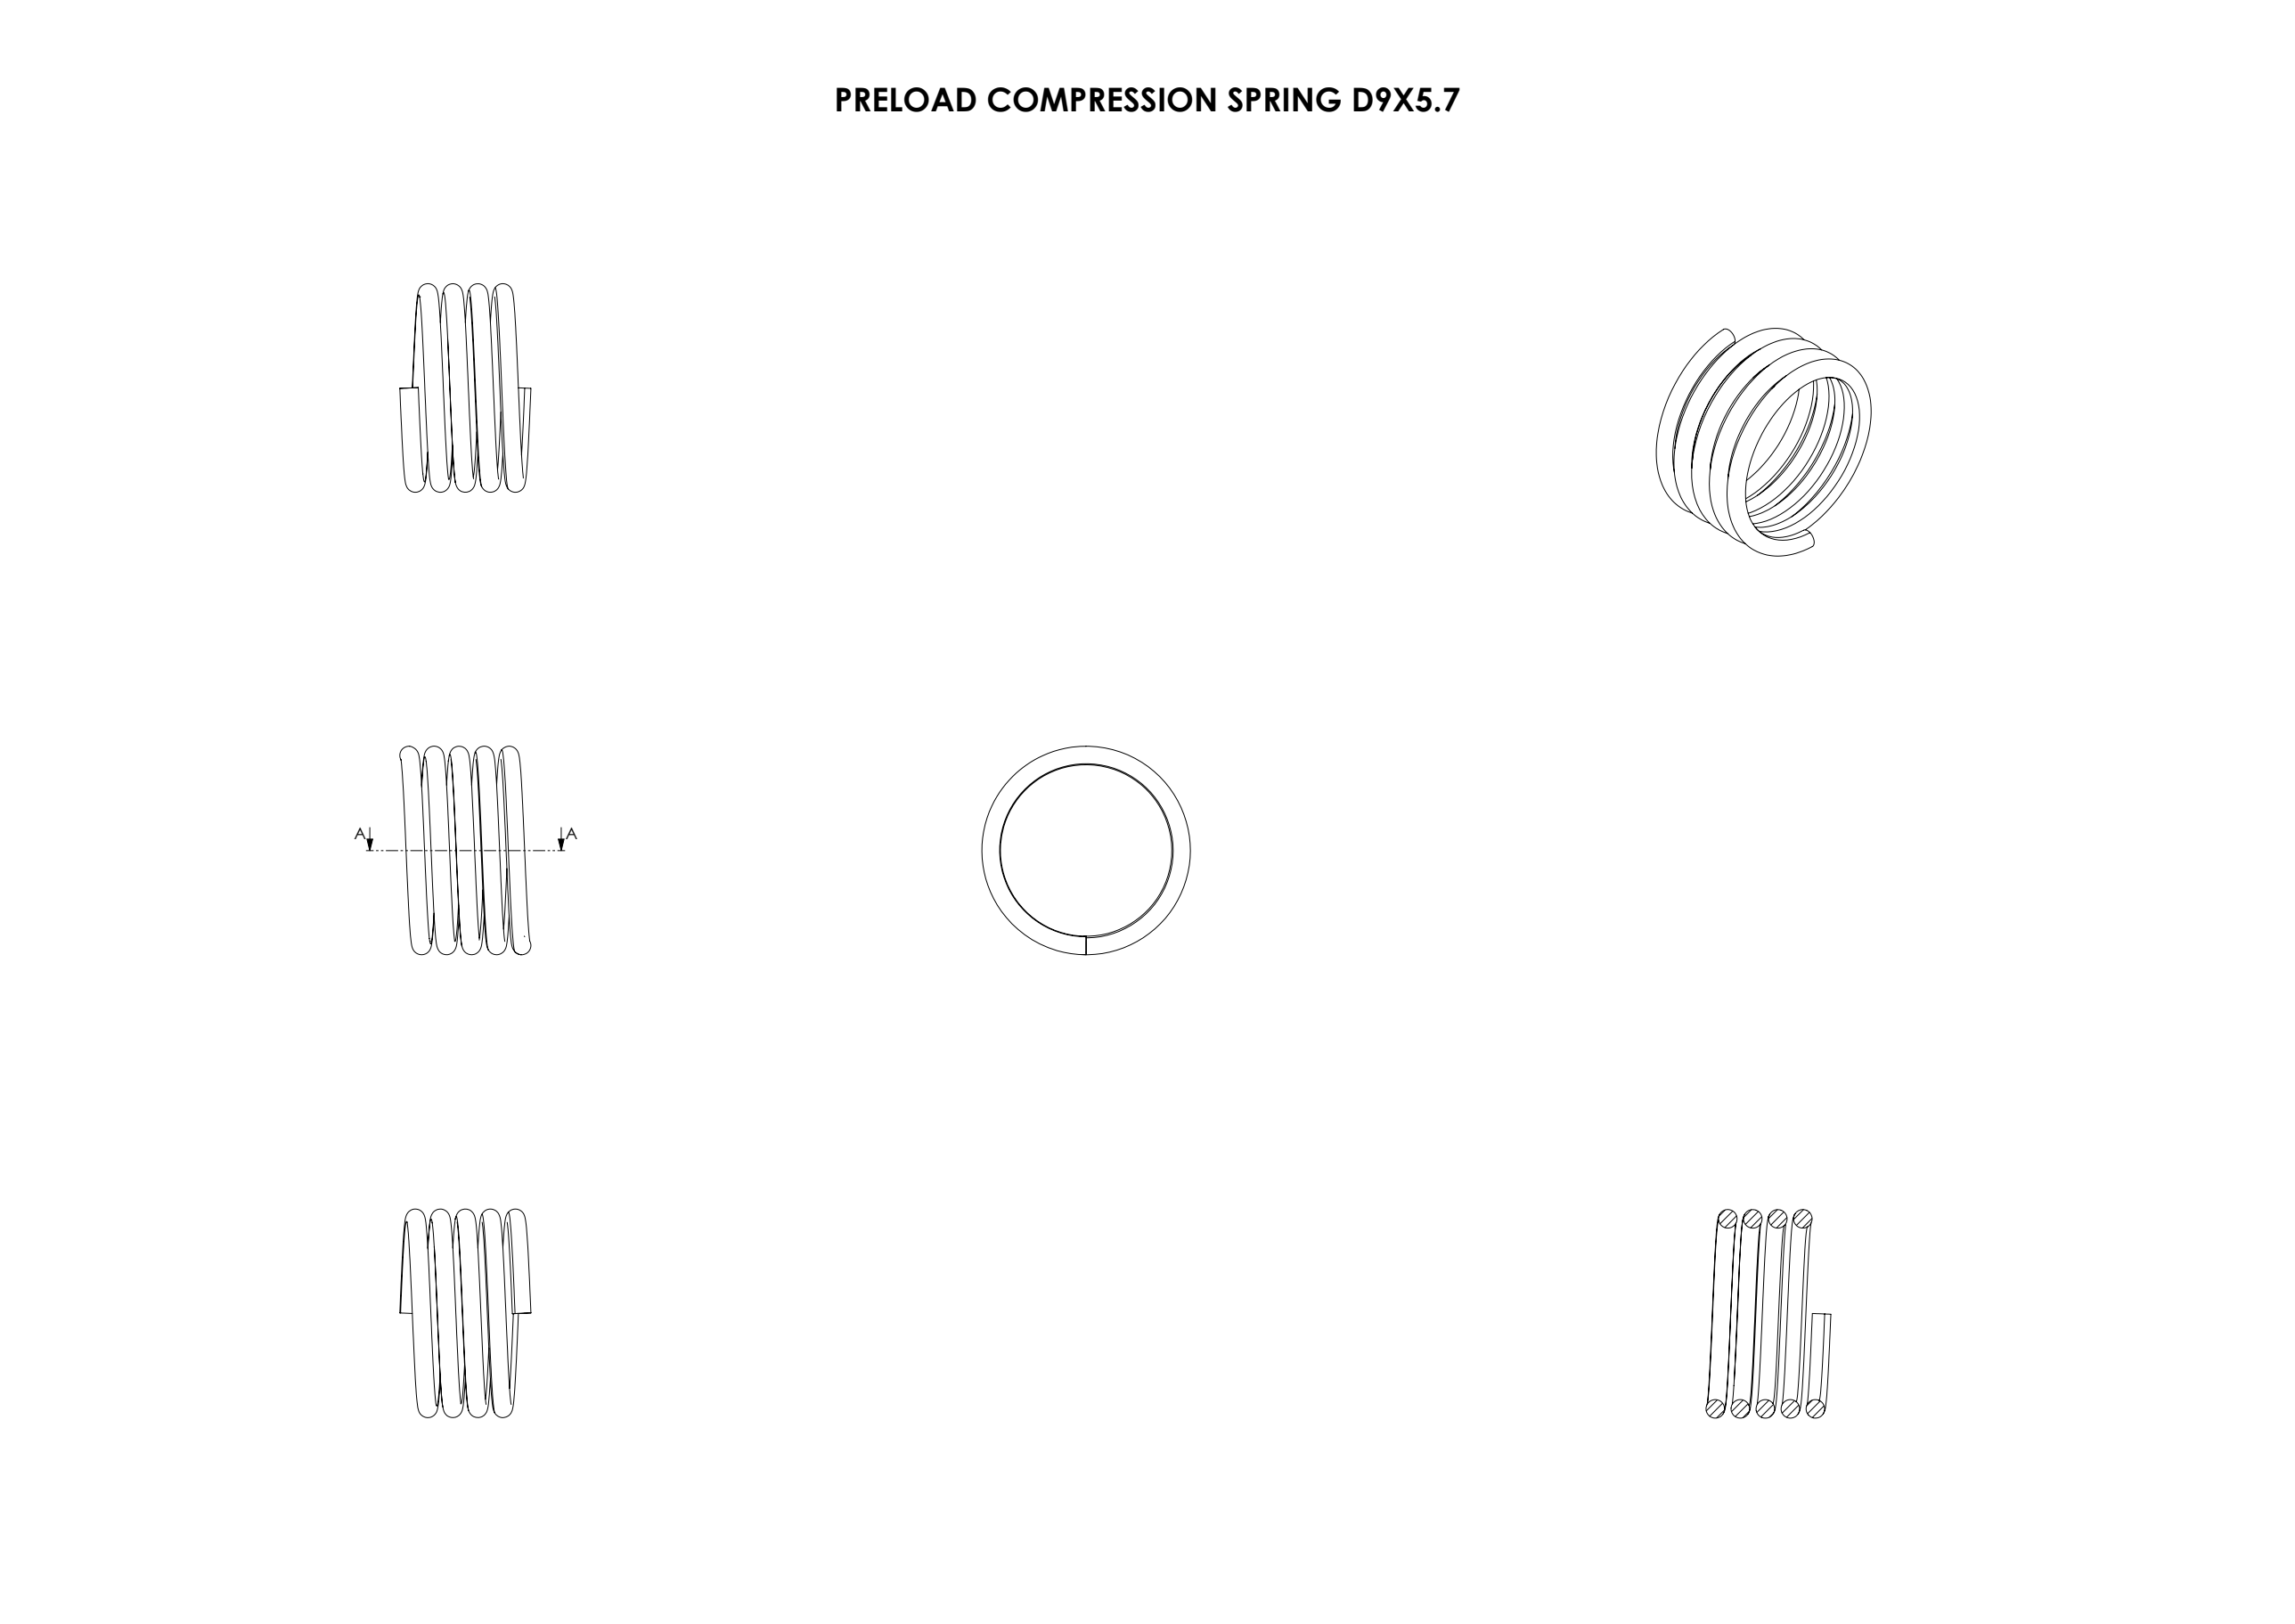
ISO-10303-21;
HEADER;
/* Generated by software containing ST-Developer
 * from STEP Tools, Inc. (www.steptools.com) 
 */

FILE_DESCRIPTION(
/* description */ (''),
/* implementation_level */ '2;1');

FILE_NAME(
/* name */ '13_Preload_Compression_Spring_D9x5.7.step',
/* time_stamp */ '2026-10-21T01:56:51-07:00',
/* author */ (''),
/* organization */ (''),
/* preprocessor_version */ 'ST-DEVELOPER v20.2',
/* originating_system */ 'Autodesk Translation Framework v15.15.0.0',
/* authorisation */ '');

FILE_SCHEMA (('AUTOMOTIVE_DESIGN { 1 0 10303 214 3 1 1 }'));
ENDSEC;

DATA;
#10=MECHANICAL_DESIGN_GEOMETRIC_PRESENTATION_REPRESENTATION('',(#279),#82384);
#241=SHAPE_REPRESENTATION_RELATIONSHIP('SRR','None',#82475,#260);
#260=ADVANCED_BREP_SHAPE_REPRESENTATION('',(#298),#82374);
#279=STYLED_ITEM('',(#82631),#298);
#298=MANIFOLD_SOLID_BREP('Body1',#30670);
#421=B_SPLINE_SURFACE_WITH_KNOTS('',3,3,((#48911,#48912,#48913,#48914,#48915,
#48916,#48917,#48918,#48919,#48920,#48921,#48922,#48923,#48924,#48925,#48926,
#48927,#48928,#48929,#48930,#48931,#48932,#48933,#48934,#48935,#48936,#48937,
#48938,#48939,#48940,#48941,#48942,#48943,#48944,#48945,#48946,#48947,#48948,
#48949,#48950,#48951,#48952,#48953,#48954,#48955,#48956,#48957,#48958,#48959,
#48960,#48961,#48962,#48963,#48964,#48965,#48966,#48967),(#48968,#48969,
#48970,#48971,#48972,#48973,#48974,#48975,#48976,#48977,#48978,#48979,#48980,
#48981,#48982,#48983,#48984,#48985,#48986,#48987,#48988,#48989,#48990,#48991,
#48992,#48993,#48994,#48995,#48996,#48997,#48998,#48999,#49000,#49001,#49002,
#49003,#49004,#49005,#49006,#49007,#49008,#49009,#49010,#49011,#49012,#49013,
#49014,#49015,#49016,#49017,#49018,#49019,#49020,#49021,#49022,#49023,#49024),
(#49025,#49026,#49027,#49028,#49029,#49030,#49031,#49032,#49033,#49034,
#49035,#49036,#49037,#49038,#49039,#49040,#49041,#49042,#49043,#49044,#49045,
#49046,#49047,#49048,#49049,#49050,#49051,#49052,#49053,#49054,#49055,#49056,
#49057,#49058,#49059,#49060,#49061,#49062,#49063,#49064,#49065,#49066,#49067,
#49068,#49069,#49070,#49071,#49072,#49073,#49074,#49075,#49076,#49077,#49078,
#49079,#49080,#49081),(#49082,#49083,#49084,#49085,#49086,#49087,#49088,
#49089,#49090,#49091,#49092,#49093,#49094,#49095,#49096,#49097,#49098,#49099,
#49100,#49101,#49102,#49103,#49104,#49105,#49106,#49107,#49108,#49109,#49110,
#49111,#49112,#49113,#49114,#49115,#49116,#49117,#49118,#49119,#49120,#49121,
#49122,#49123,#49124,#49125,#49126,#49127,#49128,#49129,#49130,#49131,#49132,
#49133,#49134,#49135,#49136,#49137,#49138),(#49139,#49140,#49141,#49142,
#49143,#49144,#49145,#49146,#49147,#49148,#49149,#49150,#49151,#49152,#49153,
#49154,#49155,#49156,#49157,#49158,#49159,#49160,#49161,#49162,#49163,#49164,
#49165,#49166,#49167,#49168,#49169,#49170,#49171,#49172,#49173,#49174,#49175,
#49176,#49177,#49178,#49179,#49180,#49181,#49182,#49183,#49184,#49185,#49186,
#49187,#49188,#49189,#49190,#49191,#49192,#49193,#49194,#49195),(#49196,
#49197,#49198,#49199,#49200,#49201,#49202,#49203,#49204,#49205,#49206,#49207,
#49208,#49209,#49210,#49211,#49212,#49213,#49214,#49215,#49216,#49217,#49218,
#49219,#49220,#49221,#49222,#49223,#49224,#49225,#49226,#49227,#49228,#49229,
#49230,#49231,#49232,#49233,#49234,#49235,#49236,#49237,#49238,#49239,#49240,
#49241,#49242,#49243,#49244,#49245,#49246,#49247,#49248,#49249,#49250,#49251,
#49252),(#49253,#49254,#49255,#49256,#49257,#49258,#49259,#49260,#49261,
#49262,#49263,#49264,#49265,#49266,#49267,#49268,#49269,#49270,#49271,#49272,
#49273,#49274,#49275,#49276,#49277,#49278,#49279,#49280,#49281,#49282,#49283,
#49284,#49285,#49286,#49287,#49288,#49289,#49290,#49291,#49292,#49293,#49294,
#49295,#49296,#49297,#49298,#49299,#49300,#49301,#49302,#49303,#49304,#49305,
#49306,#49307,#49308,#49309),(#49310,#49311,#49312,#49313,#49314,#49315,
#49316,#49317,#49318,#49319,#49320,#49321,#49322,#49323,#49324,#49325,#49326,
#49327,#49328,#49329,#49330,#49331,#49332,#49333,#49334,#49335,#49336,#49337,
#49338,#49339,#49340,#49341,#49342,#49343,#49344,#49345,#49346,#49347,#49348,
#49349,#49350,#49351,#49352,#49353,#49354,#49355,#49356,#49357,#49358,#49359,
#49360,#49361,#49362,#49363,#49364,#49365,#49366),(#49367,#49368,#49369,
#49370,#49371,#49372,#49373,#49374,#49375,#49376,#49377,#49378,#49379,#49380,
#49381,#49382,#49383,#49384,#49385,#49386,#49387,#49388,#49389,#49390,#49391,
#49392,#49393,#49394,#49395,#49396,#49397,#49398,#49399,#49400,#49401,#49402,
#49403,#49404,#49405,#49406,#49407,#49408,#49409,#49410,#49411,#49412,#49413,
#49414,#49415,#49416,#49417,#49418,#49419,#49420,#49421,#49422,#49423),
(#49424,#49425,#49426,#49427,#49428,#49429,#49430,#49431,#49432,#49433,
#49434,#49435,#49436,#49437,#49438,#49439,#49440,#49441,#49442,#49443,#49444,
#49445,#49446,#49447,#49448,#49449,#49450,#49451,#49452,#49453,#49454,#49455,
#49456,#49457,#49458,#49459,#49460,#49461,#49462,#49463,#49464,#49465,#49466,
#49467,#49468,#49469,#49470,#49471,#49472,#49473,#49474,#49475,#49476,#49477,
#49478,#49479,#49480)),.UNSPECIFIED.,.T.,.F.,.F.,(4,1,1,1,1,1,1,4),(4,1,
1,1,1,1,1,1,1,1,1,1,1,1,1,1,1,1,1,1,1,1,1,1,1,1,1,1,1,1,1,1,1,1,1,1,1,1,
1,1,1,1,1,1,1,1,1,1,1,1,1,1,1,1,4),(-3.14159265358979,-2.24399475256414,
-1.34639685153848,-0.448798950512828,0.448798950512828,1.34639685153848,
2.24399475256414,3.14159265358979),(0.,0.00892857142857143,0.0178571428571429,
0.0357142857142857,0.0535714285714286,0.0714285714285714,0.0892857142857143,
0.107142857142857,0.125,0.142857142857143,0.166666666666667,0.19047619047619,
0.214285714285714,0.232142857142857,0.25,0.267857142857143,0.285714285714286,
0.303571428571429,0.321428571428571,0.339285714285714,0.357142857142857,
0.375,0.392857142857143,0.410714285714286,0.428571428571429,0.452380952380952,
0.476190476190476,0.5,0.523809523809524,0.547619047619048,0.571428571428571,
0.595238095238095,0.619047619047619,0.642857142857143,0.666666666666667,
0.682539682539682,0.698412698412698,0.714285714285714,0.73015873015873,
0.746031746031746,0.761904761904762,0.785714285714286,0.809523809523809,
0.833333333333333,0.857142857142857,0.866071428571429,0.875,0.892857142857143,
0.910714285714286,0.928571428571429,0.946428571428571,0.964285714285714,
0.982142857142857,0.991071428571429,1.),.UNSPECIFIED.);
#1533=CIRCLE('',#32089,0.4);
#1534=CIRCLE('',#32090,0.4);
#2374=B_SPLINE_CURVE_WITH_KNOTS('',3,(#49484,#49485,#49486,#49487,#49488,
#49489,#49490,#49491,#49492,#49493,#49494,#49495,#49496,#49497,#49498,#49499,
#49500,#49501,#49502,#49503,#49504,#49505,#49506,#49507,#49508,#49509,#49510,
#49511,#49512,#49513,#49514,#49515,#49516,#49517,#49518,#49519,#49520,#49521,
#49522,#49523,#49524,#49525,#49526,#49527,#49528,#49529,#49530,#49531,#49532,
#49533,#49534,#49535,#49536,#49537,#49538,#49539,#49540),.UNSPECIFIED.,
 .F.,.F.,(4,1,1,1,1,1,1,1,1,1,1,1,1,1,1,1,1,1,1,1,1,1,1,1,1,1,1,1,1,1,1,
1,1,1,1,1,1,1,1,1,1,1,1,1,1,1,1,1,1,1,1,1,1,1,4),(0.,0.00892857142857143,
0.0178571428571429,0.0357142857142857,0.0535714285714286,0.0714285714285714,
0.0892857142857143,0.107142857142857,0.125,0.142857142857143,0.166666666666667,
0.19047619047619,0.214285714285714,0.232142857142857,0.25,0.267857142857143,
0.285714285714286,0.303571428571429,0.321428571428571,0.339285714285714,
0.357142857142857,0.375,0.392857142857143,0.410714285714286,0.428571428571429,
0.452380952380952,0.476190476190476,0.5,0.523809523809524,0.547619047619048,
0.571428571428571,0.595238095238095,0.619047619047619,0.642857142857143,
0.666666666666667,0.682539682539682,0.698412698412698,0.714285714285714,
0.73015873015873,0.746031746031746,0.761904761904762,0.785714285714286,
0.809523809523809,0.833333333333333,0.857142857142857,0.866071428571429,
0.875,0.892857142857143,0.910714285714286,0.928571428571429,0.946428571428571,
0.964285714285714,0.982142857142857,0.991071428571429,1.),.UNSPECIFIED.);
#4381=FACE_OUTER_BOUND('',#6339,.T.);
#4382=FACE_OUTER_BOUND('',#6340,.T.);
#4383=FACE_OUTER_BOUND('',#6341,.T.);
#6339=EDGE_LOOP('',(#23055,#23056,#23057,#23058));
#6340=EDGE_LOOP('',(#23059));
#6341=EDGE_LOOP('',(#23060));
#13185=VERTEX_POINT('',#49481);
#13186=VERTEX_POINT('',#49483);
#16749=EDGE_CURVE('',#13185,#13185,#1533,.T.);
#16750=EDGE_CURVE('',#13185,#13186,#2374,.T.);
#16751=EDGE_CURVE('',#13186,#13186,#1534,.T.);
#23055=ORIENTED_EDGE('',*,*,#16749,.T.);
#23056=ORIENTED_EDGE('',*,*,#16750,.T.);
#23057=ORIENTED_EDGE('',*,*,#16751,.F.);
#23058=ORIENTED_EDGE('',*,*,#16750,.F.);
#23059=ORIENTED_EDGE('',*,*,#16751,.T.);
#23060=ORIENTED_EDGE('',*,*,#16749,.F.);
#28474=PLANE('',#32091);
#28475=PLANE('',#32092);
#29709=ADVANCED_FACE('',(#4381),#421,.T.);
#29710=ADVANCED_FACE('',(#4382),#28474,.T.);
#29711=ADVANCED_FACE('',(#4383),#28475,.F.);
#30670=CLOSED_SHELL('',(#29709,#29710,#29711));
#32088=AXIS2_PLACEMENT_3D('',#48910,#36906,#36907);
#32089=AXIS2_PLACEMENT_3D('',#49482,#36908,#36909);
#32090=AXIS2_PLACEMENT_3D('',#49541,#36910,#36911);
#32091=AXIS2_PLACEMENT_3D('',#49542,#36912,#36913);
#32092=AXIS2_PLACEMENT_3D('',#49543,#36914,#36915);
#36906=DIRECTION('axis',(0.,0.,1.));
#36907=DIRECTION('refdir',(1.,0.,0.));
#36908=DIRECTION('center_axis',(0.0411785507768663,-0.00185466079691824,
0.999150082414672));
#36909=DIRECTION('ref_axis',(-0.998138206004012,0.0449556326208044,0.0412202961022186));
#36910=DIRECTION('center_axis',(0.0411785507792225,-0.00185466078915363,
-0.999150082414589));
#36911=DIRECTION('ref_axis',(-0.334687746107947,-0.94225211030106,-0.0120446352531285));
#36912=DIRECTION('center_axis',(0.0411785507792225,-0.00185466078915363,
-0.999150082414589));
#36913=DIRECTION('ref_axis',(-0.334687746107947,-0.94225211030106,-0.0120446352531285));
#36914=DIRECTION('center_axis',(0.0411785507768663,-0.00185466079691824,
0.999150082414672));
#36915=DIRECTION('ref_axis',(-0.998138206004013,0.0449556326208044,0.0412202961022186));
#48910=CARTESIAN_POINT('',(0.,0.,0.));
#48911=CARTESIAN_POINT('Ctrl Pts',(0.819255282401605,4.08201774695168,-0.0164881184408875));
#48912=CARTESIAN_POINT('Ctrl Pts',(0.833647839427758,4.08136951356852,0.332730692506625));
#48913=CARTESIAN_POINT('Ctrl Pts',(0.862424164350343,3.99464878834545,1.01269819378028));
#48914=CARTESIAN_POINT('Ctrl Pts',(0.919954808790661,3.48448113484463,2.29729435781398));
#48915=CARTESIAN_POINT('Ctrl Pts',(0.991725652203481,2.27056227452172,3.58372650506595));
#48916=CARTESIAN_POINT('Ctrl Pts',(1.07769113094686,0.253097459046851,4.2251855373779));
#48917=CARTESIAN_POINT('Ctrl Pts',(1.16347077574154,-1.81861982244698,3.81296900421478));
#48918=CARTESIAN_POINT('Ctrl Pts',(1.24907694843032,-3.42892053444273,2.45241968585354));
#48919=CARTESIAN_POINT('Ctrl Pts',(1.33450471449867,-4.17898154492915,0.486373019945627));
#48920=CARTESIAN_POINT('Ctrl Pts',(1.41975716940604,-3.88424365287751,-1.59151010962673));
#48921=CARTESIAN_POINT('Ctrl Pts',(1.51428676246171,-2.48577698688278,-3.45375961761171));
#48922=CARTESIAN_POINT('Ctrl Pts',(1.61802046319107,-0.0153163492785946,
-4.32134394881041));
#48923=CARTESIAN_POINT('Ctrl Pts',(1.73087587072984,2.67390119243303,-3.37517265531219));
#48924=CARTESIAN_POINT('Ctrl Pts',(1.8340460245136,4.05814750090039,-1.17181735141679));
#48925=CARTESIAN_POINT('Ctrl Pts',(1.92761553091683,3.9881968345771,1.13405393434499));
#48926=CARTESIAN_POINT('Ctrl Pts',(2.01165845365384,2.93784040804679,2.91554288974069));
#48927=CARTESIAN_POINT('Ctrl Pts',(2.09553292909152,1.15761277245939,3.96500388007765));
#48928=CARTESIAN_POINT('Ctrl Pts',(2.17924015408095,-0.902685284708361,
4.02211313220007));
#48929=CARTESIAN_POINT('Ctrl Pts',(2.2627817399313,-2.73048831066467,3.07746477058807));
#48930=CARTESIAN_POINT('Ctrl Pts',(2.34615886380898,-3.87072716449363,1.36987146987605));
#48931=CARTESIAN_POINT('Ctrl Pts',(2.42937324452721,-4.04253779113375,-0.672153450197734));
#48932=CARTESIAN_POINT('Ctrl Pts',(2.5124264631253,-3.20653945792688,-2.53891271248575));
#48933=CARTESIAN_POINT('Ctrl Pts',(2.59532000309479,-1.57527313865766,-3.76573008547188));
#48934=CARTESIAN_POINT('Ctrl Pts',(2.6780559376851,0.442467025625347,-4.05110137529429));
#48935=CARTESIAN_POINT('Ctrl Pts',(2.76063571470389,2.34131333359061,-3.32438634197174));
#48936=CARTESIAN_POINT('Ctrl Pts',(2.85221995159825,3.79872064908654,-1.60222299878064));
#48937=CARTESIAN_POINT('Ctrl Pts',(2.95274547399346,4.08479192723997,0.918805655449201));
#48938=CARTESIAN_POINT('Ctrl Pts',(3.06214407322622,2.6135493550915,3.25767084238896));
#48939=CARTESIAN_POINT('Ctrl Pts',(3.17128200065986,0.0126874208154328,
4.16628120635192));
#48940=CARTESIAN_POINT('Ctrl Pts',(3.2801643881585,-2.58236222387558,3.2566985796479));
#48941=CARTESIAN_POINT('Ctrl Pts',(3.38879683430733,-4.0403675070705,0.934430207343202));
#48942=CARTESIAN_POINT('Ctrl Pts',(3.49718492954501,-3.73339917040816,-1.78510203262339));
#48943=CARTESIAN_POINT('Ctrl Pts',(3.60533447778441,-1.80111124427296,-3.71502447158834));
#48944=CARTESIAN_POINT('Ctrl Pts',(3.71325145393808,0.904775445874618,-4.01918696084893));
#48945=CARTESIAN_POINT('Ctrl Pts',(3.82094203728054,3.20936283752695,-2.571197999788));
#48946=CARTESIAN_POINT('Ctrl Pts',(3.91647151249559,4.00145049915075,-0.29571072285262));
#48947=CARTESIAN_POINT('Ctrl Pts',(3.99992145777189,3.5431991882695,1.69504463314381));
#48948=CARTESIAN_POINT('Ctrl Pts',(4.07135713096102,2.45497139944041,3.06100203276521));
#48949=CARTESIAN_POINT('Ctrl Pts',(4.14270197092423,0.881853561078643,3.81799014426518));
#48950=CARTESIAN_POINT('Ctrl Pts',(4.21395799243881,-0.861429164779569,
3.81797589404032));
#48951=CARTESIAN_POINT('Ctrl Pts',(4.28512732882279,-2.42881599426564,3.0619250272124));
#48952=CARTESIAN_POINT('Ctrl Pts',(4.36805951249859,-3.69594778554289,1.47649887946172));
#48953=CARTESIAN_POINT('Ctrl Pts',(4.46270170274693,-3.96692590546529,-0.895015026539982));
#48954=CARTESIAN_POINT('Ctrl Pts',(4.56899588927351,-2.53814506387232,-3.16929534884689));
#48955=CARTESIAN_POINT('Ctrl Pts',(4.67511951925845,-0.00731392962691536,
-4.05241086380995));
#48956=CARTESIAN_POINT('Ctrl Pts',(4.75900454470091,1.98949699762205,-3.3517417086098));
#48957=CARTESIAN_POINT('Ctrl Pts',(4.82075273581193,3.02233350769069,-2.28440057824284));
#48958=CARTESIAN_POINT('Ctrl Pts',(4.87365081036613,3.65461916001154,-1.18105747976893));
#48959=CARTESIAN_POINT('Ctrl Pts',(4.93972199990629,3.88226253998919,0.430130146824839));
#48960=CARTESIAN_POINT('Ctrl Pts',(5.01892385351248,3.1862949056612,2.25227108844347));
#48961=CARTESIAN_POINT('Ctrl Pts',(5.09805405016988,1.69731476496512,3.50939368439439));
#48962=CARTESIAN_POINT('Ctrl Pts',(5.1770982730845,-0.211935388920614,3.88861454173858));
#48963=CARTESIAN_POINT('Ctrl Pts',(5.25609901422973,-2.06556469044695,3.29826074050364));
#48964=CARTESIAN_POINT('Ctrl Pts',(5.32183036241063,-3.17710297136331,2.11977728888582));
#48965=CARTESIAN_POINT('Ctrl Pts',(5.37445658284115,-3.64354521148007,0.94464387910966));
#48966=CARTESIAN_POINT('Ctrl Pts',(5.40066782824364,-3.7225043072094,0.325277046050365));
#48967=CARTESIAN_POINT('Ctrl Pts',(5.41387509844318,-3.72309915587958,0.00481785410125595));
#48968=CARTESIAN_POINT('Ctrl Pts',(0.824640136614524,4.2015762629893,-0.0164881184408875));
#48969=CARTESIAN_POINT('Ctrl Pts',(0.839431985789634,4.20091004569264,0.342419056375953));
#48970=CARTESIAN_POINT('Ctrl Pts',(0.869072200786422,4.11157275927187,1.04279181579199));
#48971=CARTESIAN_POINT('Ctrl Pts',(0.928267722148388,3.58659663339935,2.36455001110231));
#48972=CARTESIAN_POINT('Ctrl Pts',(1.00215309687483,2.33702889879683,3.68890382723956));
#48973=CARTESIAN_POINT('Ctrl Pts',(1.09062883690456,0.260587439725404,4.34897986608869));
#48974=CARTESIAN_POINT('Ctrl Pts',(1.17892287593827,-1.87177845740307,3.9247667085923));
#48975=CARTESIAN_POINT('Ctrl Pts',(1.26703196787133,-3.52913452482669,2.52439435278604));
#48976=CARTESIAN_POINT('Ctrl Pts',(1.35495625243847,-4.30109139555032,0.50094317918772));
#48977=CARTESIAN_POINT('Ctrl Pts',(1.44269582525899,-3.9977297615693,-1.63751557321081));
#48978=CARTESIAN_POINT('Ctrl Pts',(1.5399756322524,-2.5585815640104,-3.5539190962212));
#48979=CARTESIAN_POINT('Ctrl Pts',(1.64672492869982,-0.0163754272290712,
-4.44659940088065));
#48980=CARTESIAN_POINT('Ctrl Pts',(1.76283902689796,2.75044669042401,-3.47307159811878));
#48981=CARTESIAN_POINT('Ctrl Pts',(1.86897507368532,4.17436579205807,-1.20636694422441));
#48982=CARTESIAN_POINT('Ctrl Pts',(1.96522263354048,4.10238322499514,1.16541871037112));
#48983=CARTESIAN_POINT('Ctrl Pts',(2.05165710362801,3.02211393705529,2.99753313019623));
#48984=CARTESIAN_POINT('Ctrl Pts',(2.13790608656523,1.19152379694103,4.07662937239164));
#48985=CARTESIAN_POINT('Ctrl Pts',(2.22396853721079,-0.92668455854852,4.13528794998342));
#48986=CARTESIAN_POINT('Ctrl Pts',(2.30984545260645,-2.80549314624558,3.1642129683559));
#48987=CARTESIAN_POINT('Ctrl Pts',(2.39553686100961,-3.97729136934551,1.40924616985589));
#48988=CARTESIAN_POINT('Ctrl Pts',(2.48104362502894,-4.15376134490771,-0.688964949607138));
#48989=CARTESIAN_POINT('Ctrl Pts',(2.56636603958861,-3.29488852269384,-2.60662935524543));
#48990=CARTESIAN_POINT('Ctrl Pts',(2.65150601176586,-1.6194446573953,-3.86659630407993));
#48991=CARTESIAN_POINT('Ctrl Pts',(2.7364562269555,0.452274685033002,-4.15950968776552));
#48992=CARTESIAN_POINT('Ctrl Pts',(2.82123369824732,2.401520934455,-3.41344276030548));
#48993=CARTESIAN_POINT('Ctrl Pts',(2.91522208597613,3.89706826318983,-1.6460527156315));
#48994=CARTESIAN_POINT('Ctrl Pts',(3.01836404165339,4.19040693527911,0.94044790777557));
#48995=CARTESIAN_POINT('Ctrl Pts',(3.13054921535111,2.6814963714641,3.33868994257943));
#48996=CARTESIAN_POINT('Ctrl Pts',(3.24242029767871,0.0155424594777439,
4.26987430103556));
#48997=CARTESIAN_POINT('Ctrl Pts',(3.3539895659281,-2.64333786816468,3.3376826393174));
#48998=CARTESIAN_POINT('Ctrl Pts',(3.46524571947031,-4.13627311376035,0.959334384270673));
#48999=CARTESIAN_POINT('Ctrl Pts',(3.57619705361628,-3.82183356058938,-1.82432962022422));
#49000=CARTESIAN_POINT('Ctrl Pts',(3.68684681702081,-1.84478602084904,-3.79856245398834));
#49001=CARTESIAN_POINT('Ctrl Pts',(3.79720037313777,0.922021015180541,-4.10928217548828));
#49002=CARTESIAN_POINT('Ctrl Pts',(3.90726517222986,3.2771119107697,-2.62920334376493));
#49003=CARTESIAN_POINT('Ctrl Pts',(4.00483845873107,4.0857544532321,-0.305065708256623));
#49004=CARTESIAN_POINT('Ctrl Pts',(4.09002503800373,3.61790933094986,1.72702890336477));
#49005=CARTESIAN_POINT('Ctrl Pts',(4.16291899396928,2.50739659818956,3.12074066151443));
#49006=CARTESIAN_POINT('Ctrl Pts',(4.23569505179648,0.902784231955232,3.89280951201864));
#49007=CARTESIAN_POINT('Ctrl Pts',(4.30834828786622,-0.874602142649366,
3.89269192604326));
#49008=CARTESIAN_POINT('Ctrl Pts',(4.38087880591526,-2.47186195995458,3.12216898704288));
#49009=CARTESIAN_POINT('Ctrl Pts',(4.46535124680923,-3.76242506193018,1.50725518353649));
#49010=CARTESIAN_POINT('Ctrl Pts',(4.56172024478122,-4.03814548915269,-0.907329733904541));
#49011=CARTESIAN_POINT('Ctrl Pts',(4.66986044234963,-2.58427433554338,-3.22078427640133));
#49012=CARTESIAN_POINT('Ctrl Pts',(4.77776244000021,-0.0112384327514414,
-4.11841255765522));
#49013=CARTESIAN_POINT('Ctrl Pts',(4.86299326470177,2.01734328485411,-3.40624440202035));
#49014=CARTESIAN_POINT('Ctrl Pts',(4.92568672840066,3.06591863946052,-2.3226066451472));
#49015=CARTESIAN_POINT('Ctrl Pts',(4.97937885874153,3.7076520043964,-1.20271576540012));
#49016=CARTESIAN_POINT('Ctrl Pts',(5.0464263087054,3.93851483645866,0.432169333302392));
#49017=CARTESIAN_POINT('Ctrl Pts',(5.12674548922357,3.23260571308643,2.27981274817417));
#49018=CARTESIAN_POINT('Ctrl Pts',(5.2069452542926,1.72351417449459,3.55377340543451));
#49019=CARTESIAN_POINT('Ctrl Pts',(5.2870145686814,-0.210354086810664,3.93762595286232));
#49020=CARTESIAN_POINT('Ctrl Pts',(5.36698174629884,-2.08657397566065,3.34001993257469));
#49021=CARTESIAN_POINT('Ctrl Pts',(5.43350061820321,-3.21118799583293,2.14740741089702));
#49022=CARTESIAN_POINT('Ctrl Pts',(5.48669802545167,-3.68270059153974,0.959547171811996));
#49023=CARTESIAN_POINT('Ctrl Pts',(5.51320378504322,-3.76257892303397,0.333246203341611));
#49024=CARTESIAN_POINT('Ctrl Pts',(5.52654504990663,-3.76317980675502,0.00953578528314671));
#49025=CARTESIAN_POINT('Ctrl Pts',(0.721349619056559,4.4446284705926,-0.0117799836912939));
#49026=CARTESIAN_POINT('Ctrl Pts',(0.736957855041727,4.44392548365293,0.366935876306607));
#49027=CARTESIAN_POINT('Ctrl Pts',(0.768360964143123,4.34926747377125,1.10896390283271));
#49028=CARTESIAN_POINT('Ctrl Pts',(0.830966254263804,3.79399948150504,2.50685739811196));
#49029=CARTESIAN_POINT('Ctrl Pts',(0.909210267000149,2.47103126673906,3.90955883472892));
#49030=CARTESIAN_POINT('Ctrl Pts',(1.00291621006086,0.271693767768096,4.60862704115563));
#49031=CARTESIAN_POINT('Ctrl Pts',(1.0964998335884,-1.98838678064238,4.159329753954));
#49032=CARTESIAN_POINT('Ctrl Pts',(1.18992635866776,-3.74592111887884,2.67442969917082));
#49033=CARTESIAN_POINT('Ctrl Pts',(1.28320714472658,-4.56505572410638,0.527791428817508));
#49034=CARTESIAN_POINT('Ctrl Pts',(1.37633252272725,-4.24320511158861,-1.74204226726109));
#49035=CARTESIAN_POINT('Ctrl Pts',(1.47963324006593,-2.71509531029906,-3.77713627432662));
#49036=CARTESIAN_POINT('Ctrl Pts',(1.59303642701725,-0.0144100838093061,
-4.72580783762743));
#49037=CARTESIAN_POINT('Ctrl Pts',(1.71646151777425,2.92674151457479,-3.69119740428124));
#49038=CARTESIAN_POINT('Ctrl Pts',(1.82933043318807,4.44124697239644,-1.28077969442911));
#49039=CARTESIAN_POINT('Ctrl Pts',(1.93171929991264,4.36476264210786,1.24245072999059));
#49040=CARTESIAN_POINT('Ctrl Pts',(2.02369784986608,3.21525962979788,3.19218270635683));
#49041=CARTESIAN_POINT('Ctrl Pts',(2.11550244926919,1.2667206481616,4.34090326895668));
#49042=CARTESIAN_POINT('Ctrl Pts',(2.20713114238615,-0.988562626728529,
4.40343714551048));
#49043=CARTESIAN_POINT('Ctrl Pts',(2.29858133892869,-2.98941688938529,3.36936251834729));
#49044=CARTESIAN_POINT('Ctrl Pts',(2.38985139584946,-4.23760513244482,1.50010391473584));
#49045=CARTESIAN_POINT('Ctrl Pts',(2.48093895485383,-4.42565896182909,-0.73514385559243));
#49046=CARTESIAN_POINT('Ctrl Pts',(2.57184221732155,-3.51061303053924,-2.77835529581547));
#49047=CARTESIAN_POINT('Ctrl Pts',(2.66255917237085,-1.72534777250972,-4.12094012326353));
#49048=CARTESIAN_POINT('Ctrl Pts',(2.75308995897641,0.482512841602628,-4.43315431624234));
#49049=CARTESIAN_POINT('Ctrl Pts',(2.84342871960781,2.55977655442506,-3.63808847502519));
#49050=CARTESIAN_POINT('Ctrl Pts',(2.94359478029657,4.15371119436262,-1.75447635724346));
#49051=CARTESIAN_POINT('Ctrl Pts',(3.0534993425427,4.46628458035253,1.00183963908389));
#49052=CARTESIAN_POINT('Ctrl Pts',(3.17305409175693,2.85824449239317,3.55773500128709));
#49053=CARTESIAN_POINT('Ctrl Pts',(3.29225985050516,0.0173235716522711,
4.54988594670075));
#49054=CARTESIAN_POINT('Ctrl Pts',(3.4111105227762,-2.81524508966015,3.55670262369316));
#49055=CARTESIAN_POINT('Ctrl Pts',(3.52960855645907,-4.405387229637,1.02329494694289));
#49056=CARTESIAN_POINT('Ctrl Pts',(3.6477501002266,-4.07038494409819,-1.94097575854084));
#49057=CARTESIAN_POINT('Ctrl Pts',(3.76553344210117,-1.96563188563558,-4.04254830277241));
#49058=CARTESIAN_POINT('Ctrl Pts',(3.88295640499411,0.978743431351436,-4.37306760064782));
#49059=CARTESIAN_POINT('Ctrl Pts',(4.00001647488213,3.48362425976114,-2.79862452415612));
#49060=CARTESIAN_POINT('Ctrl Pts',(4.10374982384875,4.34335375479657,-0.327542203921762));
#49061=CARTESIAN_POINT('Ctrl Pts',(4.19428357469367,3.84599312218839,1.83216290559211));
#49062=CARTESIAN_POINT('Ctrl Pts',(4.27172174146588,2.66619885637548,3.31283119466691));
#49063=CARTESIAN_POINT('Ctrl Pts',(4.3489962055938,0.962215676959993,4.13258461147938));
#49064=CARTESIAN_POINT('Ctrl Pts',(4.42610940427065,-0.924394322650957,
4.13239028422168));
#49065=CARTESIAN_POINT('Ctrl Pts',(4.50306202721066,-2.61909336374746,3.31471375033465));
#49066=CARTESIAN_POINT('Ctrl Pts',(4.59265492084215,-3.98783075870693,1.60177932334117));
#49067=CARTESIAN_POINT('Ctrl Pts',(4.69476794148969,-4.27957493282873,-0.957131878749704));
#49068=CARTESIAN_POINT('Ctrl Pts',(4.80928970451843,-2.73953987979411,-3.40712746382027));
#49069=CARTESIAN_POINT('Ctrl Pts',(4.92344454247167,-0.0168010565349765,
-4.35630898735798));
#49070=CARTESIAN_POINT('Ctrl Pts',(5.01353042498076,2.12747449769232,-3.6032744047598));
#49071=CARTESIAN_POINT('Ctrl Pts',(5.07977128366408,3.23540859117732,-2.45821654233957));
#49072=CARTESIAN_POINT('Ctrl Pts',(5.13648217147255,3.9132385700417,-1.27530118138368));
#49073=CARTESIAN_POINT('Ctrl Pts',(5.20723938783248,4.15676099397256,0.450296379183357));
#49074=CARTESIAN_POINT('Ctrl Pts',(5.29195031220706,3.41204160437477,2.39903766275371));
#49075=CARTESIAN_POINT('Ctrl Pts',(5.37646206815912,1.82147811323575,3.74154376031287));
#49076=CARTESIAN_POINT('Ctrl Pts',(5.46077274553291,-0.215006596808714,
4.14549362307883));
#49077=CARTESIAN_POINT('Ctrl Pts',(5.54489246234653,-2.18888112277199,3.51672742480131));
#49078=CARTESIAN_POINT('Ctrl Pts',(5.61481604425459,-3.3708591485671,2.26269917616057));
#49079=CARTESIAN_POINT('Ctrl Pts',(5.67067535851732,-3.86597185995675,1.01536008122));
#49080=CARTESIAN_POINT('Ctrl Pts',(5.69854838705874,-3.94993232400006,0.356719058343651));
#49081=CARTESIAN_POINT('Ctrl Pts',(5.71252681611691,-3.95056190526938,0.0175485853374247));
#49082=CARTESIAN_POINT('Ctrl Pts',(0.338294245062112,4.55057569759653,0.0042037625125323));
#49083=CARTESIAN_POINT('Ctrl Pts',(0.354268648491283,4.54985621866307,0.391804253585384));
#49084=CARTESIAN_POINT('Ctrl Pts',(0.386459378345815,4.45283082043768,1.15244596626663));
#49085=CARTESIAN_POINT('Ctrl Pts',(0.450616543875562,3.88385341068114,2.58501032157865));
#49086=CARTESIAN_POINT('Ctrl Pts',(0.530955849690747,2.52591527649954,4.02565141037595));
#49087=CARTESIAN_POINT('Ctrl Pts',(0.627316019963871,0.264310635675801,
4.74491088714956));
#49088=CARTESIAN_POINT('Ctrl Pts',(0.723735630399143,-2.06432369137029,
4.28261993537111));
#49089=CARTESIAN_POINT('Ctrl Pts',(0.820158716135239,-3.87859456041539,
2.75041308513713));
#49090=CARTESIAN_POINT('Ctrl Pts',(0.916604340177546,-4.72602159109779,
0.531153832572511));
#49091=CARTESIAN_POINT('Ctrl Pts',(1.01305708152335,-4.3931659313265,-1.81989142402865));
#49092=CARTESIAN_POINT('Ctrl Pts',(1.12023653269649,-2.80816949118131,-3.9317242365496));
#49093=CARTESIAN_POINT('Ctrl Pts',(1.23813434882944,-0.000845642312135034,
-4.91906623538766));
#49094=CARTESIAN_POINT('Ctrl Pts',(1.36674602112875,3.06436157356124,-3.84215147235125));
#49095=CARTESIAN_POINT('Ctrl Pts',(1.48462403231379,4.64699863806454,-1.32534654137082));
#49096=CARTESIAN_POINT('Ctrl Pts',(1.5917660543832,4.56754799498206,1.31508654618603));
#49097=CARTESIAN_POINT('Ctrl Pts',(1.68817454439384,3.36309034412128,3.35895443333445));
#49098=CARTESIAN_POINT('Ctrl Pts',(1.78455906475243,1.31760244443516,4.56540662740121));
#49099=CARTESIAN_POINT('Ctrl Pts',(1.88091586352283,-1.05403946201403,4.63164486754336));
#49100=CARTESIAN_POINT('Ctrl Pts',(1.97723984292947,-3.16173649335291,3.54288691717697));
#49101=CARTESIAN_POINT('Ctrl Pts',(2.07352760672484,-4.47893140935848,1.57113238893729));
#49102=CARTESIAN_POINT('Ctrl Pts',(2.16977428334187,-4.67809571146175,-0.790665594289713));
#49103=CARTESIAN_POINT('Ctrl Pts',(2.26597577186357,-3.71014035199594,-2.95313903444104));
#49104=CARTESIAN_POINT('Ctrl Pts',(2.36212818012517,-1.81819297436985,-4.37651655635092));
#49105=CARTESIAN_POINT('Ctrl Pts',(2.45822704593622,0.525382903834377,-4.70837370126972));
#49106=CARTESIAN_POINT('Ctrl Pts',(2.55426812798931,2.73390242131373,-3.86353524962737));
#49107=CARTESIAN_POINT('Ctrl Pts',(2.66091177974622,4.43125636327941,-1.85846415538236));
#49108=CARTESIAN_POINT('Ctrl Pts',(2.778125747073,4.76554836922057,1.08098165568452));
#49109=CARTESIAN_POINT('Ctrl Pts',(2.90586892717749,3.04823830608109,3.81245443079));
#49110=CARTESIAN_POINT('Ctrl Pts',(3.0334755035129,0.00746606555007182,
4.87546967927499));
#49111=CARTESIAN_POINT('Ctrl Pts',(3.16093638887513,-3.03058736838478,3.81127322987509));
#49112=CARTESIAN_POINT('Ctrl Pts',(3.28824189006681,-4.73967683233644,1.09011017587669));
#49113=CARTESIAN_POINT('Ctrl Pts',(3.41538293420855,-4.38008226091659,-2.10000329693593));
#49114=CARTESIAN_POINT('Ctrl Pts',(3.54235044805458,-2.11186742976046,-4.36603149706744));
#49115=CARTESIAN_POINT('Ctrl Pts',(3.66913560141088,1.06707005130317,-4.72372043413534));
#49116=CARTESIAN_POINT('Ctrl Pts',(3.79572968394069,3.77635347593267,-3.02180133458617));
#49117=CARTESIAN_POINT('Ctrl Pts',(3.90807986203822,4.70807681195506,-0.345707133205359));
#49118=CARTESIAN_POINT('Ctrl Pts',(4.00625086823649,4.16903836543804,1.99624669567541));
#49119=CARTESIAN_POINT('Ctrl Pts',(4.09030243497979,2.88864931482185,3.60345074345437));
#49120=CARTESIAN_POINT('Ctrl Pts',(4.17425667899429,1.03751182625136,4.49424551995377));
#49121=CARTESIAN_POINT('Ctrl Pts',(4.25811096117765,-1.01398351055992,4.49423193370373));
#49122=CARTESIAN_POINT('Ctrl Pts',(4.34186270486352,-2.85847066249326,3.60451089771684));
#49123=CARTESIAN_POINT('Ctrl Pts',(4.43945045829832,-4.34951025112053,1.73889518038142));
#49124=CARTESIAN_POINT('Ctrl Pts',(4.55080259036115,-4.66822863041078,-1.0513329150146));
#49125=CARTESIAN_POINT('Ctrl Pts',(4.67582439075613,-2.98754166448033,-3.72620227444088));
#49126=CARTESIAN_POINT('Ctrl Pts',(4.80059124105991,-0.0120263346449302,
-4.76420085141347));
#49127=CARTESIAN_POINT('Ctrl Pts',(4.89915759678945,2.33414178609631,-3.94066076243851));
#49128=CARTESIAN_POINT('Ctrl Pts',(4.97167566555085,3.54709124235374,-2.68713431954456));
#49129=CARTESIAN_POINT('Ctrl Pts',(5.03378324431733,4.28942840336649,-1.39170068273366));
#49130=CARTESIAN_POINT('Ctrl Pts',(5.11132117925335,4.55644642555039,0.499203058196916));
#49131=CARTESIAN_POINT('Ctrl Pts',(5.204211387733,3.74000364932671,2.63600318529615));
#49132=CARTESIAN_POINT('Ctrl Pts',(5.29693616161317,1.99500656671931,4.10924355241873));
#49133=CARTESIAN_POINT('Ctrl Pts',(5.38950997969758,-0.240812582675891,
4.55262068051626));
#49134=CARTESIAN_POINT('Ctrl Pts',(5.48189232557165,-2.40883366006337,3.86258435496537));
#49135=CARTESIAN_POINT('Ctrl Pts',(5.55878512673359,-3.70832690498296,2.48354978245651));
#49136=CARTESIAN_POINT('Ctrl Pts',(5.62013978700551,-4.25231974581853,1.11355089098657));
#49137=CARTESIAN_POINT('Ctrl Pts',(5.65086529948741,-4.34491805581802,0.387529562643469));
#49138=CARTESIAN_POINT('Ctrl Pts',(5.66616207112364,-4.34560701456032,0.0163710261772646));
#49139=CARTESIAN_POINT('Ctrl Pts',(0.0170593592885323,4.31704107416506,
0.0170095058833432));
#49140=CARTESIAN_POINT('Ctrl Pts',(0.0322611335795961,4.31635639405152,
0.385863041260761));
#49141=CARTESIAN_POINT('Ctrl Pts',(0.0627811164807782,4.22437961039894,
1.10702759249781));
#49142=CARTESIAN_POINT('Ctrl Pts',(0.123740644702303,3.68390364811152,2.46821503884992));
#49143=CARTESIAN_POINT('Ctrl Pts',(0.200137694585886,2.39277960921485,3.83834435684185));
#49144=CARTESIAN_POINT('Ctrl Pts',(0.291937383647275,0.238467124150499,
4.52412171480303));
#49145=CARTESIAN_POINT('Ctrl Pts',(0.383934796302062,-1.98348327945548,
4.08341629079867));
#49146=CARTESIAN_POINT('Ctrl Pts',(0.476092625455518,-3.71777484054837,
2.61943491788025));
#49147=CARTESIAN_POINT('Ctrl Pts',(0.56842428847296,-4.52951306801332,0.495006553824729));
#49148=CARTESIAN_POINT('Ctrl Pts',(0.660920234839758,-4.2107917226016,-1.75962219957637));
#49149=CARTESIAN_POINT('Ctrl Pts',(0.763876444042794,-2.68873282536383,
-3.78855127791505));
#49150=CARTESIAN_POINT('Ctrl Pts',(0.87735917552732,0.0130019404539594,
-4.73992215653712));
#49151=CARTESIAN_POINT('Ctrl Pts',(1.00143747209998,2.97060794801125,-3.70215346005079));
#49152=CARTESIAN_POINT('Ctrl Pts',(1.1154269878762,4.50194744597732,-1.26897989212455));
#49153=CARTESIAN_POINT('Ctrl Pts',(1.21924908958377,4.42558239314702,1.28967440102454));
#49154=CARTESIAN_POINT('Ctrl Pts',(1.31283559471094,3.25681703771963,3.27395184877909));
#49155=CARTESIAN_POINT('Ctrl Pts',(1.40656633944771,1.26794513627352,4.44763751155047));
#49156=CARTESIAN_POINT('Ctrl Pts',(1.50043819264168,-1.04250891768418,4.51269321358057));
#49157=CARTESIAN_POINT('Ctrl Pts',(1.59444757833183,-3.09978507668561,3.45058005865305));
#49158=CARTESIAN_POINT('Ctrl Pts',(1.68859182136922,-4.38809455742526,1.52302965753274));
#49159=CARTESIAN_POINT('Ctrl Pts',(1.78286724301521,-4.58371350320302,-0.790333782115738));
#49160=CARTESIAN_POINT('Ctrl Pts',(1.87727051009661,-3.63435021507503,-2.91259494370384));
#49161=CARTESIAN_POINT('Ctrl Pts',(1.97179874248413,-1.77469819511752,-4.31235357101871));
#49162=CARTESIAN_POINT('Ctrl Pts',(2.06644688130757,0.53340573178967,-4.63973867522705));
#49163=CARTESIAN_POINT('Ctrl Pts',(2.16121394362965,2.71281770433348,-3.8066169222486));
#49164=CARTESIAN_POINT('Ctrl Pts',(2.26663623481388,4.39117481455026,-1.82494485863798));
#49165=CARTESIAN_POINT('Ctrl Pts',(2.3827596064462,4.72356161527894,1.08695595365977));
#49166=CARTESIAN_POINT('Ctrl Pts',(2.50962550191681,3.01919334092261,3.80038703978924));
#49167=CARTESIAN_POINT('Ctrl Pts',(2.63667020255104,-0.00773784804516612,
4.85999193198101));
#49168=CARTESIAN_POINT('Ctrl Pts',(2.76388543993548,-3.04038192998101,3.79913758985865));
#49169=CARTESIAN_POINT('Ctrl Pts',(2.8912606984098,-4.75154001018512,1.07720632230085));
#49170=CARTESIAN_POINT('Ctrl Pts',(3.01878711224752,-4.39221276685536,-2.12271333904207));
#49171=CARTESIAN_POINT('Ctrl Pts',(3.1464553025505,-2.112434572143,-4.40221261301575));
#49172=CARTESIAN_POINT('Ctrl Pts',(3.27425588526695,1.09179351798158,-4.7640888732722));
#49173=CARTESIAN_POINT('Ctrl Pts',(3.40217948205457,3.83027103061875,-3.04548218475403));
#49174=CARTESIAN_POINT('Ctrl Pts',(3.51598938618772,4.7752036557919,-0.334962986231444));
#49175=CARTESIAN_POINT('Ctrl Pts',(3.61563973232771,4.22849780113868,2.04242980680349));
#49176=CARTESIAN_POINT('Ctrl Pts',(3.70109729466062,2.92698374082993,3.67674162607492));
#49177=CARTESIAN_POINT('Ctrl Pts',(3.78659509245201,1.04198382964828,4.58426838084057));
#49178=CARTESIAN_POINT('Ctrl Pts',(3.87212990675981,-1.05062940346987,4.58464289114657));
#49179=CARTESIAN_POINT('Ctrl Pts',(3.95769867440709,-2.93530142451636,3.67594696906703));
#49180=CARTESIAN_POINT('Ctrl Pts',(4.05756489439709,-4.46149605353647,1.7670832262665));
#49181=CARTESIAN_POINT('Ctrl Pts',(4.1717454215982,-4.78942536463651,-1.09384432241825));
#49182=CARTESIAN_POINT('Ctrl Pts',(4.30025111609553,-3.06306433763481,-3.84395647764373));
#49183=CARTESIAN_POINT('Ctrl Pts',(4.42879998759059,0.00225573918968807,
-4.91468643030986));
#49184=CARTESIAN_POINT('Ctrl Pts',(4.5305942867175,2.4256086471289,-4.06511079601246));
#49185=CARTESIAN_POINT('Ctrl Pts',(4.60560876665858,3.68042867344509,-2.76847280341322));
#49186=CARTESIAN_POINT('Ctrl Pts',(4.66991088188852,4.44905704578208,-1.42732745616853));
#49187=CARTESIAN_POINT('Ctrl Pts',(4.75029250165825,4.72630844924892,0.532881291021042));
#49188=CARTESIAN_POINT('Ctrl Pts',(4.84675818745935,3.87892864485845,2.75210127777632));
#49189=CARTESIAN_POINT('Ctrl Pts',(4.94321603172176,2.0639903822995,4.28511445138593));
#49190=CARTESIAN_POINT('Ctrl Pts',(5.03968552854927,-0.265786119546311,
4.74757649013579));
#49191=CARTESIAN_POINT('Ctrl Pts',(5.13610992605831,-2.52891273917334,4.02793579977318));
#49192=CARTESIAN_POINT('Ctrl Pts',(5.21651607630675,-3.88799657674959,2.58610912462865));
#49193=CARTESIAN_POINT('Ctrl Pts',(5.28073297925971,-4.45751297641237,1.15222839320222));
#49194=CARTESIAN_POINT('Ctrl Pts',(5.31295628255007,-4.55464067477421,0.390818592699824));
#49195=CARTESIAN_POINT('Ctrl Pts',(5.32894534279131,-4.5553608138399,0.00286247099432417));
#49196=CARTESIAN_POINT('Ctrl Pts',(-0.000509373030547474,3.92021534661009,
0.016996973047247));
#49197=CARTESIAN_POINT('Ctrl Pts',(0.0133655849277437,3.91959042562335,
0.353656839069412));
#49198=CARTESIAN_POINT('Ctrl Pts',(0.0410178057586762,3.83628172595668,
1.00706848486642));
#49199=CARTESIAN_POINT('Ctrl Pts',(0.0964473712623517,3.3449812065841,2.24480055647181));
#49200=CARTESIAN_POINT('Ctrl Pts',(0.165833000914959,2.17209893003467,3.48910168092513));
#49201=CARTESIAN_POINT('Ctrl Pts',(0.249299786414105,0.213616043118768,
4.11301832351545));
#49202=CARTESIAN_POINT('Ctrl Pts',(0.332952618295147,-1.80695501753449,
3.71214532456504));
#49203=CARTESIAN_POINT('Ctrl Pts',(0.416802497335945,-3.38495223229509,
2.38039261819367));
#49204=CARTESIAN_POINT('Ctrl Pts',(0.500846500139207,-4.12396088271141,
0.446611903120177));
#49205=CARTESIAN_POINT('Ctrl Pts',(0.585087885198009,-3.83383487106712,
-1.60680296233244));
#49206=CARTESIAN_POINT('Ctrl Pts',(0.678908855398844,-2.4469602145113,-3.45582042752092));
#49207=CARTESIAN_POINT('Ctrl Pts',(0.78239581946303,0.0166703941746675,
-4.32374610526772));
#49208=CARTESIAN_POINT('Ctrl Pts',(0.895646446224181,2.71635016747082,-3.37695733163609));
#49209=CARTESIAN_POINT('Ctrl Pts',(0.999787586550202,4.11575032209256,-1.15422710837935));
#49210=CARTESIAN_POINT('Ctrl Pts',(1.09472345355387,4.04616602639483,1.18546806705486));
#49211=CARTESIAN_POINT('Ctrl Pts',(1.18036859245895,2.97675618213071,3.00148026190969));
#49212=CARTESIAN_POINT('Ctrl Pts',(1.26621705771563,1.155248892265,4.07666825088898));
#49213=CARTESIAN_POINT('Ctrl Pts',(1.35226925935515,-0.962745675997109,
4.13654259389504));
#49214=CARTESIAN_POINT('Ctrl Pts',(1.43852556730039,-2.85047653482757,3.16223962035245));
#49215=CARTESIAN_POINT('Ctrl Pts',(1.52498617068693,-4.03385922256971,1.39214156439959));
#49216=CARTESIAN_POINT('Ctrl Pts',(1.61165124607536,-4.21395408979635,-0.734463165223846));
#49217=CARTESIAN_POINT('Ctrl Pts',(1.69852082762757,-3.34060056023991,-2.68748353854695));
#49218=CARTESIAN_POINT('Ctrl Pts',(1.78559486750465,-1.62775490667668,-3.97709376117724));
#49219=CARTESIAN_POINT('Ctrl Pts',(1.87287344377062,0.500587977333086,-4.27928334792637));
#49220=CARTESIAN_POINT('Ctrl Pts',(1.96035587732167,2.51259896961598,-3.51047090069615));
#49221=CARTESIAN_POINT('Ctrl Pts',(2.05778526152882,4.06396467869906,-1.6792876022321));
#49222=CARTESIAN_POINT('Ctrl Pts',(2.16524726584212,4.37226319720578,1.0153436549924));
#49223=CARTESIAN_POINT('Ctrl Pts',(2.2828395210483,2.79318044202061,3.53087293178842));
#49224=CARTESIAN_POINT('Ctrl Pts',(2.40079070809031,-0.0168285977474749,
4.51542105142518));
#49225=CARTESIAN_POINT('Ctrl Pts',(2.51909864959676,-2.83743776879735,3.52966478818611));
#49226=CARTESIAN_POINT('Ctrl Pts',(2.63776186062134,-4.43231756105859,0.994362843096609));
#49227=CARTESIAN_POINT('Ctrl Pts',(2.75677778921884,-4.09788532816048,-1.99212131743342));
#49228=CARTESIAN_POINT('Ctrl Pts',(2.87614384522742,-1.96701233519621,-4.12407406978207));
#49229=CARTESIAN_POINT('Ctrl Pts',(2.99585707630498,1.03434971847348,-4.46399782820216));
#49230=CARTESIAN_POINT('Ctrl Pts',(3.11591416505015,3.60498437698043,-2.85193723841394));
#49231=CARTESIAN_POINT('Ctrl Pts',(3.22293457137712,4.49439067358845,-0.303368192450996));
#49232=CARTESIAN_POINT('Ctrl Pts',(3.31679611001667,3.97978943060175,1.9360373994789));
#49233=CARTESIAN_POINT('Ctrl Pts',(3.39739730622727,2.7524658458149,3.47765530299832));
#49234=CARTESIAN_POINT('Ctrl Pts',(3.47814554446175,0.972308519013181,4.33504755156959));
#49235=CARTESIAN_POINT('Ctrl Pts',(3.55903990182147,-1.00678432949211,4.33571435385092));
#49236=CARTESIAN_POINT('Ctrl Pts',(3.64007911331806,-2.79183322033623,3.47538186734198));
#49237=CARTESIAN_POINT('Ctrl Pts',(3.73479255980622,-4.23956446318879,1.66526560265338));
#49238=CARTESIAN_POINT('Ctrl Pts',(3.84327171133281,-4.55205389252981,-1.05267677488261));
#49239=CARTESIAN_POINT('Ctrl Pts',(3.96562611564225,-2.90933219122212,-3.67175612600794));
#49240=CARTESIAN_POINT('Ctrl Pts',(4.08828871140458,0.0152883107737241,
-4.69457325075005));
#49241=CARTESIAN_POINT('Ctrl Pts',(4.18563699424379,2.33312265754483,-3.8829464124187));
#49242=CARTESIAN_POINT('Ctrl Pts',(4.25748715092105,3.53511437004692,-2.64104529091489));
#49243=CARTESIAN_POINT('Ctrl Pts',(4.31912870973056,4.27199921354012,-1.35544035073423));
#49244=CARTESIAN_POINT('Ctrl Pts',(4.39628211340819,4.53851738355101,0.525971082460842));
#49245=CARTESIAN_POINT('Ctrl Pts',(4.48903104290479,3.72425076863922,2.65992095145394));
#49246=CARTESIAN_POINT('Ctrl Pts',(4.58193549181756,1.97650556376007,4.13676409759574));
#49247=CARTESIAN_POINT('Ctrl Pts',(4.67500541351684,-0.271152556122982,
4.5835619815803));
#49248=CARTESIAN_POINT('Ctrl Pts',(4.76821030596407,-2.45874208118696,3.88828759969444));
#49249=CARTESIAN_POINT('Ctrl Pts',(4.84603932740361,-3.77474566277566,2.49302437023683));
#49250=CARTESIAN_POINT('Ctrl Pts',(4.90832676369923,-4.32719027071689,1.10223497733668));
#49251=CARTESIAN_POINT('Ctrl Pts',(4.93956556049856,-4.42134796182669,0.364085063305676));
#49252=CARTESIAN_POINT('Ctrl Pts',(4.95509803681809,-4.42204753658693,-0.0127925756858374));
#49253=CARTESIAN_POINT('Ctrl Pts',(0.298096584279089,3.65836109017721,0.00420428892078251));
#49254=CARTESIAN_POINT('Ctrl Pts',(0.311087334711855,3.6577759934437,0.319409878254403));
#49255=CARTESIAN_POINT('Ctrl Pts',(0.336830084091236,3.5802354464982,0.927709628550148));
#49256=CARTESIAN_POINT('Ctrl Pts',(0.38855260702266,3.12183104328619,2.08266824732869));
#49257=CARTESIAN_POINT('Ctrl Pts',(0.453129934636734,2.02971933680628,3.24042531085447));
#49258=CARTESIAN_POINT('Ctrl Pts',(0.530755063824667,0.208415697693674,
3.8205922887506));
#49259=CARTESIAN_POINT('Ctrl Pts',(0.608414396037071,-1.66745393285822,
3.44786535315643));
#49260=CARTESIAN_POINT('Ctrl Pts',(0.686159436538254,-3.13032413522546,
2.21294951308035));
#49261=CARTESIAN_POINT('Ctrl Pts',(0.763972879863645,-3.81423765920946,
0.422321925736774));
#49262=CARTESIAN_POINT('Ctrl Pts',(0.84186845439323,-3.54566782855519,-1.47634282001782));
#49263=CARTESIAN_POINT('Ctrl Pts',(0.928510023393671,-2.26460758686192,
-3.18369230311773));
#49264=CARTESIAN_POINT('Ctrl Pts',(1.02393926290267,0.00745279667992231,
-3.98343126373423));
#49265=CARTESIAN_POINT('Ctrl Pts',(1.1282088165072,2.49279512049407,-3.11107079600691));
#49266=CARTESIAN_POINT('Ctrl Pts',(1.22394778855269,3.77880815931524,-1.06735588227691));
#49267=CARTESIAN_POINT('Ctrl Pts',(1.31111514094575,3.71461026876317,1.08086001346169));
#49268=CARTESIAN_POINT('Ctrl Pts',(1.3896723008585,2.73349922536098,2.7464657129172));
#49269=CARTESIAN_POINT('Ctrl Pts',(1.46833905161798,1.06424073934361,3.73150146410114));
#49270=CARTESIAN_POINT('Ctrl Pts',(1.54711899544478,-0.874769694920365,
3.78609161644686));
#49271=CARTESIAN_POINT('Ctrl Pts',(1.62601619609109,-2.60134983389898,2.89471971378898));
#49272=CARTESIAN_POINT('Ctrl Pts',(1.70503355230775,-3.68268674678379,1.27689142569084));
#49273=CARTESIAN_POINT('Ctrl Pts',(1.78417499391135,-3.8469551181542,-0.6651138286791));
#49274=CARTESIAN_POINT('Ctrl Pts',(1.86344387042269,-3.04984922963428,-2.44717700797688));
#49275=CARTESIAN_POINT('Ctrl Pts',(1.94284316920819,-1.48787263639168,-3.62298369274466));
#49276=CARTESIAN_POINT('Ctrl Pts',(2.02237693622473,0.451629060530175,-3.89819852788527));
#49277=CARTESIAN_POINT('Ctrl Pts',(2.10204759676506,2.28391860618936,-3.1979016042206));
#49278=CARTESIAN_POINT('Ctrl Pts',(2.19072686284899,3.69583592175625,-1.53107534941479));
#49279=CARTESIAN_POINT('Ctrl Pts',(2.28847866353304,3.97600385511532,0.920104709516196));
#49280=CARTESIAN_POINT('Ctrl Pts',(2.39537928379895,2.54026942442417,3.20676446315769));
#49281=CARTESIAN_POINT('Ctrl Pts',(2.50254921833245,-0.0129562004679963,
4.10110737239459));
#49282=CARTESIAN_POINT('Ctrl Pts',(2.60999586145542,-2.57453765912131,3.20567216837469));
#49283=CARTESIAN_POINT('Ctrl Pts',(2.71772516765194,-4.02232258005484,0.903913813484832));
#49284=CARTESIAN_POINT('Ctrl Pts',(2.82574372839834,-3.71867938979836,-1.80657721613234));
#49285=CARTESIAN_POINT('Ctrl Pts',(2.93405757815297,-1.78506235042054,-3.74105574559891));
#49286=CARTESIAN_POINT('Ctrl Pts',(3.04267271783813,0.938031464050205,-4.04941214503227));
#49287=CARTESIAN_POINT('Ctrl Pts',(3.15159502061989,3.27021991188957,-2.58686956509611));
#49288=CARTESIAN_POINT('Ctrl Pts',(3.24869195571493,4.07715622206919,-0.274641703989928));
#49289=CARTESIAN_POINT('Ctrl Pts',(3.33385675064398,3.6102629295096,1.75726838594271));
#49290=CARTESIAN_POINT('Ctrl Pts',(3.40699786221515,2.49655157382426,3.15620212552146));
#49291=CARTESIAN_POINT('Ctrl Pts',(3.48028345483719,0.880944659700569,3.93437721261743));
#49292=CARTESIAN_POINT('Ctrl Pts',(3.55371422038057,-0.915536983185619,
3.93501794003845));
#49293=CARTESIAN_POINT('Ctrl Pts',(3.62729125737481,-2.53622425264173,3.15395432305343));
#49294=CARTESIAN_POINT('Ctrl Pts',(3.71330261507569,-3.8509806770859,1.51019720414124));
#49295=CARTESIAN_POINT('Ctrl Pts',(3.8118527186074,-4.13505336346601,-0.958902703289102));
#49296=CARTESIAN_POINT('Ctrl Pts',(3.92305859063978,-2.64222932727816,-3.33943426601281));
#49297=CARTESIAN_POINT('Ctrl Pts',(4.03460899727506,0.0172906347131659,
-4.26987015966603));
#49298=CARTESIAN_POINT('Ctrl Pts',(4.12319413503313,2.12653084069738,-3.53152596583768));
#49299=CARTESIAN_POINT('Ctrl Pts',(4.18860565230255,3.22082638065193,-2.40094424117363));
#49300=CARTESIAN_POINT('Ctrl Pts',(4.24473809079781,3.89186716862466,-1.23025202544185));
#49301=CARTESIAN_POINT('Ctrl Pts',(4.31502966074825,4.13478863470262,0.483742163642918));
#49302=CARTESIAN_POINT('Ctrl Pts',(4.39957589386275,3.39268989860514,2.429083429048));
#49303=CARTESIAN_POINT('Ctrl Pts',(4.48432451794297,1.79854838577187,3.77622697986339));
#49304=CARTESIAN_POINT('Ctrl Pts',(4.5692686183663,-0.252936245272161,4.18443079336503));
#49305=CARTESIAN_POINT('Ctrl Pts',(4.65442518287259,-2.25140394373808,3.5490997128701));
#49306=CARTESIAN_POINT('Ctrl Pts',(4.72553786073744,-3.45425595710783,2.27452643733581));
#49307=CARTESIAN_POINT('Ctrl Pts',(4.78256122142649,-3.95993018611354,1.0012669710165));
#49308=CARTESIAN_POINT('Ctrl Pts',(4.81107750552547,-4.04587113521165,0.327446493022771));
#49309=CARTESIAN_POINT('Ctrl Pts',(4.82534909064748,-4.0465139200796,-0.0188370740532776));
#49310=CARTESIAN_POINT('Ctrl Pts',(0.688956982238612,3.72989859436059,-0.011771676272502));
#49311=CARTESIAN_POINT('Ctrl Pts',(0.702174766109974,3.7293032721575,0.308942617826199));
#49312=CARTESIAN_POINT('Ctrl Pts',(0.728412419797738,3.65025149910867,0.928927699894124));
#49313=CARTESIAN_POINT('Ctrl Pts',(0.781055770698673,3.18356680884235,2.1044162778148));
#49314=CARTESIAN_POINT('Ctrl Pts',(0.846674620528363,2.07353195281602,3.28052198629612));
#49315=CARTESIAN_POINT('Ctrl Pts',(0.925372417292195,0.226915654958949,
3.86816221327804));
#49316=CARTESIAN_POINT('Ctrl Pts',(1.0039282373004,-1.67046670484249,3.49061937856621));
#49317=CARTESIAN_POINT('Ctrl Pts',(1.08239262224571,-3.14650150602498,2.24387354628045));
#49318=CARTESIAN_POINT('Ctrl Pts',(1.16074810104558,-3.83465270230634,0.440602979531981));
#49319=CARTESIAN_POINT('Ctrl Pts',(1.23900844652084,-3.56429950374443,-1.46684219978431));
#49320=CARTESIAN_POINT('Ctrl Pts',(1.32585707942573,-2.27966928390904,-3.17791782495388));
#49321=CARTESIAN_POINT('Ctrl Pts',(1.42126320702305,-0.00774635499684935,
-3.9763100078759));
#49322=CARTESIAN_POINT('Ctrl Pts',(1.5251889897962,2.46889842538329,-3.1055672655037));
#49323=CARTESIAN_POINT('Ctrl Pts',(1.62032386985681,3.74579076667661,-1.07411530102224));
#49324=CARTESIAN_POINT('Ctrl Pts',(1.70671299419631,3.68153000413254,1.05483485686011));
#49325=CARTESIAN_POINT('Ctrl Pts',(1.78439233771942,2.71093422500403,2.70156674187247));
#49326=CARTESIAN_POINT('Ctrl Pts',(1.86200496845593,1.06376581310854,3.67292919184799));
#49327=CARTESIAN_POINT('Ctrl Pts',(1.93955458075406,-0.844971763668853,
3.72613393319396));
#49328=CARTESIAN_POINT('Ctrl Pts',(2.01704603660621,-2.54054699924709,2.85016942977958));
#49329=CARTESIAN_POINT('Ctrl Pts',(2.09448268075612,-3.59981265404682,1.2644088722943));
#49330=CARTESIAN_POINT('Ctrl Pts',(2.17186924701519,-3.75991607911409,-0.634585005549751));
#49331=CARTESIAN_POINT('Ctrl Pts',(2.24920986959975,-2.98172066966817,-2.37309080416439));
#49332=CARTESIAN_POINT('Ctrl Pts',(2.32650817304572,-1.46075735861725,-3.5173780157574));
#49333=CARTESIAN_POINT('Ctrl Pts',(2.4037704539101,0.423440863053585,-3.78422132593972));
#49334=CARTESIAN_POINT('Ctrl Pts',(2.48099742993376,2.19935922972781,-3.10493127396526));
#49335=CARTESIAN_POINT('Ctrl Pts',(2.56677463084692,3.56466710193294,-1.49224467784406));
#49336=CARTESIAN_POINT('Ctrl Pts',(2.66109148663689,3.83389443421792,0.872997558466858));
#49337=CARTESIAN_POINT('Ctrl Pts',(2.76395230037421,2.45138388800358,3.07261614748915));
#49338=CARTESIAN_POINT('Ctrl Pts',(2.86678959686819,0.000962930291893762,
3.92967379273786));
#49339=CARTESIAN_POINT('Ctrl Pts',(2.96961058667187,-2.44999053829016,3.0716577741312));
#49340=CARTESIAN_POINT('Ctrl Pts',(3.07242986170307,-3.83085160241301,0.874160218469037));
#49341=CARTESIAN_POINT('Ctrl Pts',(3.17525621245274,-3.5406642117419,-1.70597889374842));
#49342=CARTESIAN_POINT('Ctrl Pts',(3.27810003269075,-1.70389003181941,-3.54201749378549));
#49343=CARTESIAN_POINT('Ctrl Pts',(3.38097100851841,0.875408995607918,-3.83303032919846));
#49344=CARTESIAN_POINT('Ctrl Pts',(3.48387834482028,3.07828851197773,-2.45029862200831));
#49345=CARTESIAN_POINT('Ctrl Pts',(3.57539602828975,3.83808495585644,-0.270620622306617));
#49346=CARTESIAN_POINT('Ctrl Pts',(3.65551391848674,3.39850167651178,1.64079042729728));
#49347=CARTESIAN_POINT('Ctrl Pts',(3.72421465191342,2.35218871393199,2.95467125124523));
#49348=CARTESIAN_POINT('Ctrl Pts',(3.79294539429065,0.836823541180858,3.68423759790819));
#49349=CARTESIAN_POINT('Ctrl Pts',(3.86171128648602,-0.845569294720187,
3.6845686834364));
#49350=CARTESIAN_POINT('Ctrl Pts',(3.9305160372789,-2.36105179514293,2.95390454763975));
#49351=CARTESIAN_POINT('Ctrl Pts',(4.01083890816804,-3.58862834578777,1.41862728882207));
#49352=CARTESIAN_POINT('Ctrl Pts',(4.10270010008198,-3.85262944454734,-0.88313055241628));
#49353=CARTESIAN_POINT('Ctrl Pts',(4.20615878865277,-2.4630265539622,-3.09744279594199));
#49354=CARTESIAN_POINT('Ctrl Pts',(4.30973054597676,0.00668693977155496,
-3.96049481183038));
#49355=CARTESIAN_POINT('Ctrl Pts',(4.39182398199372,1.96125111015289,-3.27568322468014));
#49356=CARTESIAN_POINT('Ctrl Pts',(4.45237494972608,2.9741864942725,-2.2290598638584));
#49357=CARTESIAN_POINT('Ctrl Pts',(4.50430190138047,3.59493532071667,-1.14601631965969));
#49358=CARTESIAN_POINT('Ctrl Pts',(4.56925693234196,3.81916629261384,0.4379350138335));
#49359=CARTESIAN_POINT('Ctrl Pts',(4.64728728639836,3.13397091050645,2.23339295261525));
#49360=CARTESIAN_POINT('Ctrl Pts',(4.72541311711678,1.66418205411997,3.47494711303392));
#49361=CARTESIAN_POINT('Ctrl Pts',(4.80361529922962,-0.224728631862202,
3.85074359773365));
#49362=CARTESIAN_POINT('Ctrl Pts',(4.88195040442182,-2.06287164850845,3.26576977045013));
#49363=CARTESIAN_POINT('Ctrl Pts',(4.94724603874465,-3.16747854887194,2.09537568929752));
#49364=CARTESIAN_POINT('Ctrl Pts',(4.99963868315035,-3.63192116122577,0.925462967583616));
#49365=CARTESIAN_POINT('Ctrl Pts',(5.02574333679671,-3.71055096761041,0.308604734669394));
#49366=CARTESIAN_POINT('Ctrl Pts',(5.03890131113639,-3.71114359602036,-0.0106583500463774));
#49367=CARTESIAN_POINT('Ctrl Pts',(0.813870428188686,3.96245923091406,-0.0164881184408875));
#49368=CARTESIAN_POINT('Ctrl Pts',(0.827863881435175,3.96182897296034,0.323046899201097));
#49369=CARTESIAN_POINT('Ctrl Pts',(0.855776576686915,3.8777235191813,0.98261372822563));
#49370=CARTESIAN_POINT('Ctrl Pts',(0.91164293979103,3.38235777450735,2.23005863274043));
#49371=CARTESIAN_POINT('Ctrl Pts',(0.981299333783199,2.20407781698023,3.47855069743377));
#49372=CARTESIAN_POINT('Ctrl Pts',(1.06475475796298,0.245591313523208,4.10137579394894));
#49373=CARTESIAN_POINT('Ctrl Pts',(1.14801995745261,-1.76546201737438,3.70113724609284));
#49374=CARTESIAN_POINT('Ctrl Pts',(1.23112334588228,-3.3286789257896,2.38040969948328));
#49375=CARTESIAN_POINT('Ctrl Pts',(1.31405425162276,-4.0568214497295,0.471783311416064));
#49376=CARTESIAN_POINT('Ctrl Pts',(1.39682007324284,-3.77068607508619,-1.54548516328751));
#49377=CARTESIAN_POINT('Ctrl Pts',(1.48859751335545,-2.41293504528005,-3.3535345600583));
#49378=CARTESIAN_POINT('Ctrl Pts',(1.58932060338395,-0.0141931238132137,
-4.1959578414747));
#49379=CARTESIAN_POINT('Ctrl Pts',(1.69891363944235,2.59730954355204,-3.2771941918542));
#49380=CARTESIAN_POINT('Ctrl Pts',(1.79911717211155,3.94178755900518,-1.13723469292121));
#49381=CARTESIAN_POINT('Ctrl Pts',(1.89001020184871,3.87387138983037,1.10266716450794));
#49382=CARTESIAN_POINT('Ctrl Pts',(1.97166092482987,2.85344269161481,2.83344742015103));
#49383=CARTESIAN_POINT('Ctrl Pts',(2.05316121208527,1.12364269113143,3.85321962107559));
#49384=CARTESIAN_POINT('Ctrl Pts',(2.13451307741901,-0.878658896837783,
3.90875659364244));
#49385=CARTESIAN_POINT('Ctrl Pts',(2.21571945417949,-2.65536261814589,2.99056101462381));
#49386=CARTESIAN_POINT('Ctrl Pts',(2.2967823085229,-3.76397021259743,1.33041373899585));
#49387=CARTESIAN_POINT('Ctrl Pts',(2.37770464847043,-3.93109025436271,-0.655327951595781));
#49388=CARTESIAN_POINT('Ctrl Pts',(2.45848894616092,-3.11798970322431,-2.47107411872514));
#49389=CARTESIAN_POINT('Ctrl Pts',(2.539138236748,-1.53095692651357,-3.6646976699462));
#49390=CARTESIAN_POINT('Ctrl Pts',(2.61965150239195,0.43254661592197,-3.94244977897841));
#49391=CARTESIAN_POINT('Ctrl Pts',(2.70003978500417,2.28096457989066,-3.2351055267086));
#49392=CARTESIAN_POINT('Ctrl Pts',(2.78921497281684,3.70005464083461,-1.55832357099016));
#49393=CARTESIAN_POINT('Ctrl Pts',(2.88713754483823,3.978871723082,0.897304502209273));
#49394=CARTESIAN_POINT('Ctrl Pts',(2.99373926382005,2.54539755561737,3.1764149602916));
#49395=CARTESIAN_POINT('Ctrl Pts',(3.10013487511961,0.0100260539871462,
4.06239810401769));
#49396=CARTESIAN_POINT('Ctrl Pts',(3.20633868411026,-2.52115841647006,3.17542686994721));
#49397=CARTESIAN_POINT('Ctrl Pts',(3.31234811237552,-3.94408155000773,0.90944188237858));
#49398=CARTESIAN_POINT('Ctrl Pts',(3.41817428538941,-3.6446229361879,-1.74571659991173));
#49399=CARTESIAN_POINT('Ctrl Pts',(3.52382459568201,-1.75722515420472,-3.63111700668246));
#49400=CARTESIAN_POINT('Ctrl Pts',(3.62930813345658,0.887450966770746,-3.92861999578969));
#49401=CARTESIAN_POINT('Ctrl Pts',(3.73463542446446,3.14148071884394,-2.51269203574673));
#49402=CARTESIAN_POINT('Ctrl Pts',(3.82812092232632,3.91670767970764,-0.286048650138266));
#49403=CARTESIAN_POINT('Ctrl Pts',(3.90982285467911,3.46818164980758,1.66298970973192));
#49404=CARTESIAN_POINT('Ctrl Pts',(3.97979345533908,2.40232887286283,3.0009094587564));
#49405=CARTESIAN_POINT('Ctrl Pts',(4.0497099280914,0.860827997743688,3.74279364024213));
#49406=CARTESIAN_POINT('Ctrl Pts',(4.11956952823211,-0.848223352254005,
3.74285099046553));
#49407=CARTESIAN_POINT('Ctrl Pts',(4.18937342077798,-2.38551844241705,3.00143347916426));
#49408=CARTESIAN_POINT('Ctrl Pts',(4.27074480521005,-3.62886084584353,1.44594609859824));
#49409=CARTESIAN_POINT('Ctrl Pts',(4.36368118378899,-3.89527620214059,-0.882569356349999));
#49410=CARTESIAN_POINT('Ctrl Pts',(4.46811929683045,-2.49174100886108,-3.11716551782941));
#49411=CARTESIAN_POINT('Ctrl Pts',(4.57247822032509,-0.00337846350186114,
-3.98594899624739));
#49412=CARTESIAN_POINT('Ctrl Pts',(4.65503336657386,1.96170059971088,-3.29661664499807));
#49413=CARTESIAN_POINT('Ctrl Pts',(4.71582271106075,2.9784869170383,-2.24591417407558));
#49414=CARTESIAN_POINT('Ctrl Pts',(4.76791393631401,3.60111877586318,-1.15944268096052));
#49415=CARTESIAN_POINT('Ctrl Pts',(4.83301893094167,3.82552050348602,0.428030004985985));
#49416=CARTESIAN_POINT('Ctrl Pts',(4.91110192413723,3.1395319735366,2.2243674028123));
#49417=CARTESIAN_POINT('Ctrl Pts',(4.98916391106651,1.67086400618948,3.46453264131029));
#49418=CARTESIAN_POINT('Ctrl Pts',(5.06718831755995,-0.213604995253956,
3.83895695068989));
#49419=CARTESIAN_POINT('Ctrl Pts',(5.14521889040735,-2.04438566721443,3.25600753491638));
#49420=CARTESIAN_POINT('Ctrl Pts',(5.21018829958173,-3.14309383374398,2.09139171932537));
#49421=CARTESIAN_POINT('Ctrl Pts',(5.26222496048943,-3.60433678749298,0.929455512264779));
#49422=CARTESIAN_POINT('Ctrl Pts',(5.28813860325278,-3.68242999458204,0.317144549177678));
#49423=CARTESIAN_POINT('Ctrl Pts',(5.30120514697973,-3.68301850500413,9.99229193651664E-5));
#49424=CARTESIAN_POINT('Ctrl Pts',(0.819255282401605,4.08201774695168,-0.0164881184408875));
#49425=CARTESIAN_POINT('Ctrl Pts',(0.833647839427758,4.08136951356852,0.332730692506625));
#49426=CARTESIAN_POINT('Ctrl Pts',(0.862424164350343,3.99464878834545,1.01269819378028));
#49427=CARTESIAN_POINT('Ctrl Pts',(0.919954808790661,3.48448113484463,2.29729435781398));
#49428=CARTESIAN_POINT('Ctrl Pts',(0.991725652203481,2.27056227452172,3.58372650506595));
#49429=CARTESIAN_POINT('Ctrl Pts',(1.07769113094686,0.253097459046851,4.2251855373779));
#49430=CARTESIAN_POINT('Ctrl Pts',(1.16347077574154,-1.81861982244698,3.81296900421478));
#49431=CARTESIAN_POINT('Ctrl Pts',(1.24907694843032,-3.42892053444273,2.45241968585354));
#49432=CARTESIAN_POINT('Ctrl Pts',(1.33450471449867,-4.17898154492915,0.486373019945627));
#49433=CARTESIAN_POINT('Ctrl Pts',(1.41975716940604,-3.8842436528775,-1.59151010962673));
#49434=CARTESIAN_POINT('Ctrl Pts',(1.51428676246171,-2.48577698688278,-3.45375961761171));
#49435=CARTESIAN_POINT('Ctrl Pts',(1.61802046319107,-0.0153163492785947,
-4.32134394881041));
#49436=CARTESIAN_POINT('Ctrl Pts',(1.73087587072984,2.67390119243303,-3.37517265531219));
#49437=CARTESIAN_POINT('Ctrl Pts',(1.8340460245136,4.05814750090038,-1.17181735141679));
#49438=CARTESIAN_POINT('Ctrl Pts',(1.92761553091683,3.9881968345771,1.134053934345));
#49439=CARTESIAN_POINT('Ctrl Pts',(2.01165845365384,2.93784040804679,2.91554288974069));
#49440=CARTESIAN_POINT('Ctrl Pts',(2.09553292909152,1.15761277245939,3.96500388007765));
#49441=CARTESIAN_POINT('Ctrl Pts',(2.17924015408095,-0.902685284708361,
4.02211313220007));
#49442=CARTESIAN_POINT('Ctrl Pts',(2.2627817399313,-2.73048831066467,3.07746477058807));
#49443=CARTESIAN_POINT('Ctrl Pts',(2.34615886380898,-3.87072716449363,1.36987146987605));
#49444=CARTESIAN_POINT('Ctrl Pts',(2.42937324452721,-4.04253779113375,-0.672153450197734));
#49445=CARTESIAN_POINT('Ctrl Pts',(2.5124264631253,-3.20653945792688,-2.53891271248575));
#49446=CARTESIAN_POINT('Ctrl Pts',(2.59532000309479,-1.57527313865766,-3.76573008547188));
#49447=CARTESIAN_POINT('Ctrl Pts',(2.6780559376851,0.442467025625347,-4.05110137529429));
#49448=CARTESIAN_POINT('Ctrl Pts',(2.76063571470389,2.34131333359061,-3.32438634197174));
#49449=CARTESIAN_POINT('Ctrl Pts',(2.85221995159825,3.79872064908654,-1.60222299878064));
#49450=CARTESIAN_POINT('Ctrl Pts',(2.95274547399346,4.08479192723997,0.918805655449201));
#49451=CARTESIAN_POINT('Ctrl Pts',(3.06214407322622,2.6135493550915,3.25767084238896));
#49452=CARTESIAN_POINT('Ctrl Pts',(3.17128200065986,0.0126874208154326,
4.16628120635192));
#49453=CARTESIAN_POINT('Ctrl Pts',(3.2801643881585,-2.58236222387558,3.2566985796479));
#49454=CARTESIAN_POINT('Ctrl Pts',(3.38879683430733,-4.0403675070705,0.934430207343202));
#49455=CARTESIAN_POINT('Ctrl Pts',(3.49718492954501,-3.73339917040816,-1.78510203262339));
#49456=CARTESIAN_POINT('Ctrl Pts',(3.60533447778441,-1.80111124427296,-3.71502447158834));
#49457=CARTESIAN_POINT('Ctrl Pts',(3.71325145393808,0.904775445874618,-4.01918696084893));
#49458=CARTESIAN_POINT('Ctrl Pts',(3.82094203728053,3.20936283752695,-2.571197999788));
#49459=CARTESIAN_POINT('Ctrl Pts',(3.91647151249559,4.00145049915075,-0.29571072285262));
#49460=CARTESIAN_POINT('Ctrl Pts',(3.99992145777189,3.54319918826949,1.69504463314381));
#49461=CARTESIAN_POINT('Ctrl Pts',(4.07135713096102,2.45497139944041,3.06100203276521));
#49462=CARTESIAN_POINT('Ctrl Pts',(4.14270197092423,0.881853561078642,3.81799014426518));
#49463=CARTESIAN_POINT('Ctrl Pts',(4.21395799243881,-0.861429164779569,
3.81797589404032));
#49464=CARTESIAN_POINT('Ctrl Pts',(4.28512732882279,-2.42881599426564,3.0619250272124));
#49465=CARTESIAN_POINT('Ctrl Pts',(4.36805951249859,-3.69594778554289,1.47649887946172));
#49466=CARTESIAN_POINT('Ctrl Pts',(4.46270170274693,-3.96692590546529,-0.895015026539982));
#49467=CARTESIAN_POINT('Ctrl Pts',(4.56899588927351,-2.53814506387232,-3.16929534884689));
#49468=CARTESIAN_POINT('Ctrl Pts',(4.67511951925845,-0.00731392962691536,
-4.05241086380995));
#49469=CARTESIAN_POINT('Ctrl Pts',(4.75900454470091,1.98949699762205,-3.3517417086098));
#49470=CARTESIAN_POINT('Ctrl Pts',(4.82075273581193,3.02233350769069,-2.28440057824284));
#49471=CARTESIAN_POINT('Ctrl Pts',(4.87365081036613,3.65461916001154,-1.18105747976893));
#49472=CARTESIAN_POINT('Ctrl Pts',(4.93972199990629,3.88226253998919,0.430130146824839));
#49473=CARTESIAN_POINT('Ctrl Pts',(5.01892385351248,3.1862949056612,2.25227108844347));
#49474=CARTESIAN_POINT('Ctrl Pts',(5.09805405016988,1.69731476496512,3.50939368439439));
#49475=CARTESIAN_POINT('Ctrl Pts',(5.1770982730845,-0.211935388920614,3.88861454173858));
#49476=CARTESIAN_POINT('Ctrl Pts',(5.25609901422973,-2.06556469044695,3.29826074050364));
#49477=CARTESIAN_POINT('Ctrl Pts',(5.32183036241063,-3.17710297136331,2.11977728888582));
#49478=CARTESIAN_POINT('Ctrl Pts',(5.37445658284115,-3.64354521148007,0.94464387910966));
#49479=CARTESIAN_POINT('Ctrl Pts',(5.40066782824364,-3.7225043072094,0.325277046050365));
#49480=CARTESIAN_POINT('Ctrl Pts',(5.41387509844318,-3.72309915587958,0.00481785410125593));
#49481=CARTESIAN_POINT('',(0.819255282401605,4.08201774695168,-0.0164881184408875));
#49482=CARTESIAN_POINT('Origin',(0.42,4.1,-3.04061776853425E-19));
#49483=CARTESIAN_POINT('',(5.41387509844318,-3.72309915587958,0.00481785410125595));
#49484=CARTESIAN_POINT('Ctrl Pts',(0.819255282401605,4.08201774695168,-0.0164881184408875));
#49485=CARTESIAN_POINT('Ctrl Pts',(0.833647839427758,4.08136951356852,0.332730692506625));
#49486=CARTESIAN_POINT('Ctrl Pts',(0.862424164350343,3.99464878834545,1.01269819378028));
#49487=CARTESIAN_POINT('Ctrl Pts',(0.919954808790661,3.48448113484463,2.29729435781398));
#49488=CARTESIAN_POINT('Ctrl Pts',(0.991725652203481,2.27056227452172,3.58372650506595));
#49489=CARTESIAN_POINT('Ctrl Pts',(1.07769113094686,0.253097459046851,4.2251855373779));
#49490=CARTESIAN_POINT('Ctrl Pts',(1.16347077574154,-1.81861982244698,3.81296900421478));
#49491=CARTESIAN_POINT('Ctrl Pts',(1.24907694843032,-3.42892053444273,2.45241968585354));
#49492=CARTESIAN_POINT('Ctrl Pts',(1.33450471449867,-4.17898154492915,0.486373019945627));
#49493=CARTESIAN_POINT('Ctrl Pts',(1.41975716940604,-3.8842436528775,-1.59151010962673));
#49494=CARTESIAN_POINT('Ctrl Pts',(1.51428676246171,-2.48577698688278,-3.45375961761171));
#49495=CARTESIAN_POINT('Ctrl Pts',(1.61802046319107,-0.0153163492785947,
-4.32134394881041));
#49496=CARTESIAN_POINT('Ctrl Pts',(1.73087587072984,2.67390119243303,-3.37517265531219));
#49497=CARTESIAN_POINT('Ctrl Pts',(1.8340460245136,4.05814750090038,-1.17181735141679));
#49498=CARTESIAN_POINT('Ctrl Pts',(1.92761553091683,3.9881968345771,1.134053934345));
#49499=CARTESIAN_POINT('Ctrl Pts',(2.01165845365384,2.93784040804679,2.91554288974069));
#49500=CARTESIAN_POINT('Ctrl Pts',(2.09553292909152,1.15761277245939,3.96500388007765));
#49501=CARTESIAN_POINT('Ctrl Pts',(2.17924015408095,-0.902685284708361,
4.02211313220007));
#49502=CARTESIAN_POINT('Ctrl Pts',(2.2627817399313,-2.73048831066467,3.07746477058807));
#49503=CARTESIAN_POINT('Ctrl Pts',(2.34615886380898,-3.87072716449363,1.36987146987605));
#49504=CARTESIAN_POINT('Ctrl Pts',(2.42937324452721,-4.04253779113375,-0.672153450197734));
#49505=CARTESIAN_POINT('Ctrl Pts',(2.5124264631253,-3.20653945792688,-2.53891271248575));
#49506=CARTESIAN_POINT('Ctrl Pts',(2.59532000309479,-1.57527313865766,-3.76573008547188));
#49507=CARTESIAN_POINT('Ctrl Pts',(2.6780559376851,0.442467025625347,-4.05110137529429));
#49508=CARTESIAN_POINT('Ctrl Pts',(2.76063571470389,2.34131333359061,-3.32438634197174));
#49509=CARTESIAN_POINT('Ctrl Pts',(2.85221995159825,3.79872064908654,-1.60222299878064));
#49510=CARTESIAN_POINT('Ctrl Pts',(2.95274547399346,4.08479192723997,0.918805655449201));
#49511=CARTESIAN_POINT('Ctrl Pts',(3.06214407322622,2.6135493550915,3.25767084238896));
#49512=CARTESIAN_POINT('Ctrl Pts',(3.17128200065986,0.0126874208154326,
4.16628120635192));
#49513=CARTESIAN_POINT('Ctrl Pts',(3.2801643881585,-2.58236222387558,3.2566985796479));
#49514=CARTESIAN_POINT('Ctrl Pts',(3.38879683430733,-4.0403675070705,0.934430207343202));
#49515=CARTESIAN_POINT('Ctrl Pts',(3.49718492954501,-3.73339917040816,-1.78510203262339));
#49516=CARTESIAN_POINT('Ctrl Pts',(3.60533447778441,-1.80111124427296,-3.71502447158834));
#49517=CARTESIAN_POINT('Ctrl Pts',(3.71325145393808,0.904775445874618,-4.01918696084893));
#49518=CARTESIAN_POINT('Ctrl Pts',(3.82094203728053,3.20936283752695,-2.571197999788));
#49519=CARTESIAN_POINT('Ctrl Pts',(3.91647151249559,4.00145049915075,-0.29571072285262));
#49520=CARTESIAN_POINT('Ctrl Pts',(3.99992145777189,3.54319918826949,1.69504463314381));
#49521=CARTESIAN_POINT('Ctrl Pts',(4.07135713096102,2.45497139944041,3.06100203276521));
#49522=CARTESIAN_POINT('Ctrl Pts',(4.14270197092423,0.881853561078642,3.81799014426518));
#49523=CARTESIAN_POINT('Ctrl Pts',(4.21395799243881,-0.861429164779569,
3.81797589404032));
#49524=CARTESIAN_POINT('Ctrl Pts',(4.28512732882279,-2.42881599426564,3.0619250272124));
#49525=CARTESIAN_POINT('Ctrl Pts',(4.36805951249859,-3.69594778554289,1.47649887946172));
#49526=CARTESIAN_POINT('Ctrl Pts',(4.46270170274693,-3.96692590546529,-0.895015026539982));
#49527=CARTESIAN_POINT('Ctrl Pts',(4.56899588927351,-2.53814506387232,-3.16929534884689));
#49528=CARTESIAN_POINT('Ctrl Pts',(4.67511951925845,-0.00731392962691536,
-4.05241086380995));
#49529=CARTESIAN_POINT('Ctrl Pts',(4.75900454470091,1.98949699762205,-3.3517417086098));
#49530=CARTESIAN_POINT('Ctrl Pts',(4.82075273581193,3.02233350769069,-2.28440057824284));
#49531=CARTESIAN_POINT('Ctrl Pts',(4.87365081036613,3.65461916001154,-1.18105747976893));
#49532=CARTESIAN_POINT('Ctrl Pts',(4.93972199990629,3.88226253998919,0.430130146824839));
#49533=CARTESIAN_POINT('Ctrl Pts',(5.01892385351248,3.1862949056612,2.25227108844347));
#49534=CARTESIAN_POINT('Ctrl Pts',(5.09805405016988,1.69731476496512,3.50939368439439));
#49535=CARTESIAN_POINT('Ctrl Pts',(5.1770982730845,-0.211935388920614,3.88861454173858));
#49536=CARTESIAN_POINT('Ctrl Pts',(5.25609901422973,-2.06556469044695,3.29826074050364));
#49537=CARTESIAN_POINT('Ctrl Pts',(5.32183036241063,-3.17710297136331,2.11977728888582));
#49538=CARTESIAN_POINT('Ctrl Pts',(5.37445658284115,-3.64354521148007,0.94464387910966));
#49539=CARTESIAN_POINT('Ctrl Pts',(5.40066782824364,-3.7225043072094,0.325277046050365));
#49540=CARTESIAN_POINT('Ctrl Pts',(5.41387509844318,-3.72309915587958,0.00481785410125593));
#49541=CARTESIAN_POINT('Origin',(5.28,-4.1,4.54497550705923E-15));
#49542=CARTESIAN_POINT('Origin',(5.28,-4.1,4.54497550705923E-15));
#49543=CARTESIAN_POINT('Origin',(0.42,4.1,-3.04061776853425E-19));
#82353=UNCERTAINTY_MEASURE_WITH_UNIT(LENGTH_MEASURE(0.01),#82385,
'DISTANCE_ACCURACY_VALUE',
'Maximum model space distance between geometric entities at asserted c
onnectivities');
#82363=UNCERTAINTY_MEASURE_WITH_UNIT(LENGTH_MEASURE(0.01),#82385,
'DISTANCE_ACCURACY_VALUE',
'Maximum model space distance between geometric entities at asserted c
onnectivities');
#82374=(
GEOMETRIC_REPRESENTATION_CONTEXT(3)
GLOBAL_UNCERTAINTY_ASSIGNED_CONTEXT((#82353))
GLOBAL_UNIT_ASSIGNED_CONTEXT((#82385,#82387,#82388))
REPRESENTATION_CONTEXT('','3D')
);
#82384=(
GEOMETRIC_REPRESENTATION_CONTEXT(3)
GLOBAL_UNCERTAINTY_ASSIGNED_CONTEXT((#82363))
GLOBAL_UNIT_ASSIGNED_CONTEXT((#82385,#82387,#82388))
REPRESENTATION_CONTEXT('','3D')
);
#82385=(
LENGTH_UNIT()
NAMED_UNIT(*)
SI_UNIT(.MILLI.,.METRE.)
);
#82387=(
NAMED_UNIT(*)
PLANE_ANGLE_UNIT()
SI_UNIT($,.RADIAN.)
);
#82388=(
NAMED_UNIT(*)
SI_UNIT($,.STERADIAN.)
SOLID_ANGLE_UNIT()
);
#82399=SHAPE_DEFINITION_REPRESENTATION(#82419,#82475);
#82419=PRODUCT_DEFINITION_SHAPE('',$,#82496);
#82475=SHAPE_REPRESENTATION('',(#32088),#82374);
#82485=PRODUCT_DEFINITION_CONTEXT('part definition',#82547,'design');
#82496=PRODUCT_DEFINITION('2026-10-20-12-38-24-156',
'13_Preload_Compression_Spring_D9x5.7',#82516,#82485);
#82516=PRODUCT_DEFINITION_FORMATION('',$,#82559);
#82547=APPLICATION_CONTEXT(
'Core Data for Automotive Mechanical Design Process');
#82548=PRODUCT_CONTEXT('part definition',#82547,'mechanical');
#82559=PRODUCT('2026-10-20-12-38-24-156',
'13_Preload_Compression_Spring_D9x5.7',$,(#82548));
#82625=COLOUR_RGB('Grey',0.48,0.52,0.57);
#82626=FILL_AREA_STYLE_COLOUR('',#82625);
#82627=FILL_AREA_STYLE('',(#82626));
#82628=SURFACE_STYLE_FILL_AREA(#82627);
#82629=SURFACE_SIDE_STYLE('',(#82628));
#82630=SURFACE_STYLE_USAGE(.BOTH.,#82629);
#82631=PRESENTATION_STYLE_ASSIGNMENT((#82630));
ENDSEC;
END-ISO-10303-21;
